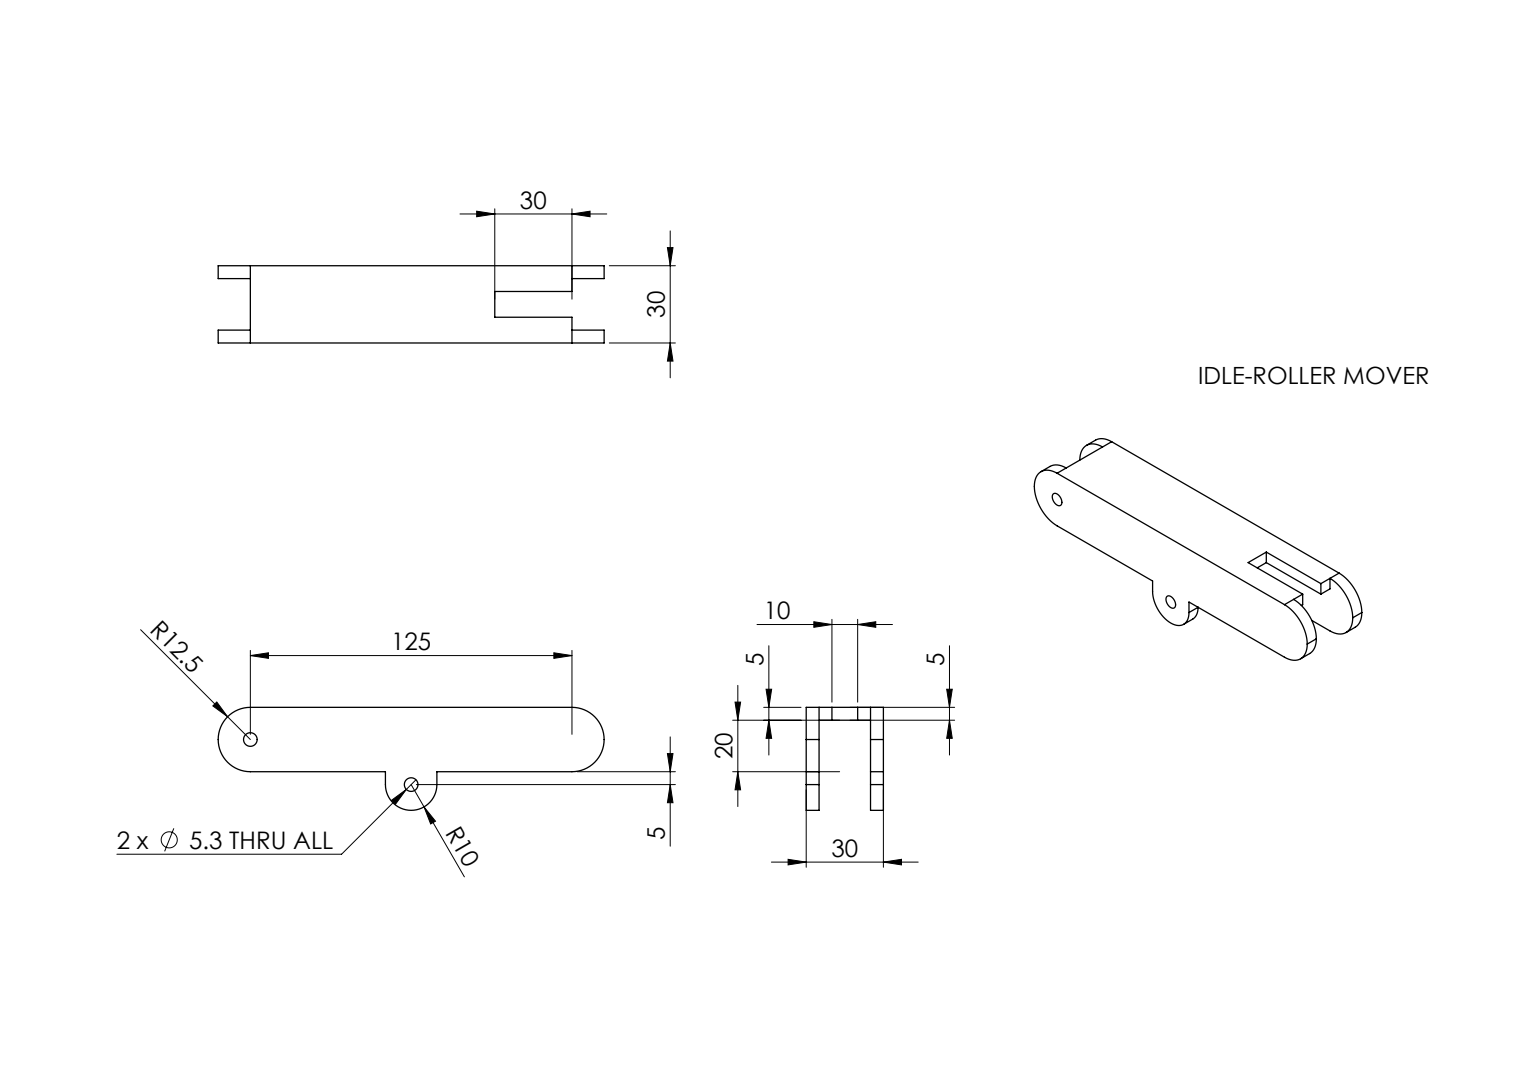
ISO-10303-21;
HEADER;
FILE_DESCRIPTION (('STEP AP214'),
    '1' );
FILE_NAME ('idle-roller mover.step',
    '2026-10-25T07:12:54',
    ( '' ),
    ( '' ),
    'SwSTEP 2.0',
    'SolidWorks 2026',
    '' );
FILE_SCHEMA (( 'AUTOMOTIVE_DESIGN' ));
ENDSEC;

DATA;
#13=CARTESIAN_POINT ( 'NONE',  ( 62.49999999999998579, 40.00000000000001421, 0.000000000000000000 ) ) ;
#53=PLANE ( 'NONE',  #5492 ) ;
#59=AXIS2_PLACEMENT_3D ( 'NONE', #3052, #893, #11418 ) ;
#61=DIRECTION ( 'NONE',  ( -1.000000000000000000, 0.000000000000000000, 0.000000000000000000 ) ) ;
#77=ORIENTED_EDGE ( 'NONE', *, *, #7381, .F. ) ;
#79=ORIENTED_EDGE ( 'NONE', *, *, #8111, .F. ) ;
#81=EDGE_CURVE ( 'NONE', #6144, #12887, #9290, .T. ) ;
#85=DIRECTION ( 'NONE',  ( 1.000000000000000000, -0.000000000000000000, 0.000000000000000000 ) ) ;
#94=ADVANCED_FACE ( 'NONE', ( #8455 ), #6331, .F. ) ;
#97=ADVANCED_FACE ( 'NONE', ( #1883, #8329, #2085 ), #7362, .T. ) ;
#98=DIRECTION ( 'NONE',  ( 0.000000000000000000, -1.000000000000000000, 0.000000000000000000 ) ) ;
#115=ORIENTED_EDGE ( 'NONE', *, *, #9892, .T. ) ;
#157=ADVANCED_FACE ( 'NONE', ( #8524 ), #11972, .T. ) ;
#164=ORIENTED_EDGE ( 'NONE', *, *, #12600, .T. ) ;
#165=CARTESIAN_POINT ( 'NONE',  ( -9.999999999999996447, 0.000000000000000000, 9.999999999999998224 ) ) ;
#166=ORIENTED_EDGE ( 'NONE', *, *, #5950, .F. ) ;
#173=DIRECTION ( 'NONE',  ( 1.000000000000000000, 0.000000000000000000, 0.000000000000000000 ) ) ;
#177=FACE_OUTER_BOUND ( 'NONE', #6171, .T. ) ;
#178=VERTEX_POINT ( 'NONE', #7689 ) ;
#182=FACE_OUTER_BOUND ( 'NONE', #2923, .T. ) ;
#199=ORIENTED_EDGE ( 'NONE', *, *, #13522, .F. ) ;
#200=CARTESIAN_POINT ( 'NONE',  ( 32.49999999999998579, 40.00000000000001421, -4.999999999999996447 ) ) ;
#212=ORIENTED_EDGE ( 'NONE', *, *, #12682, .T. ) ;
#219=FACE_BOUND ( 'NONE', #1402, .T. ) ;
#220=CARTESIAN_POINT ( 'NONE',  ( -74.99999999999997158, 20.00000000000001421, 15.00000000000000000 ) ) ;
#234=ORIENTED_EDGE ( 'NONE', *, *, #2081, .F. ) ;
#244=DIRECTION ( 'NONE',  ( 0.000000000000000000, -0.000000000000000000, 1.000000000000000000 ) ) ;
#245=VERTEX_POINT ( 'NONE', #4504 ) ;
#247=ORIENTED_EDGE ( 'NONE', *, *, #4058, .T. ) ;
#256=AXIS2_PLACEMENT_3D ( 'NONE', #2457, #12077, #2596 ) ;
#262=AXIS2_PLACEMENT_3D ( 'NONE', #4018, #5829, #10026 ) ;
#266=ADVANCED_FACE ( 'NONE', ( #8732 ), #10661, .F. ) ;
#267=EDGE_CURVE ( 'NONE', #10003, #9221, #8792, .T. ) ;
#304=CARTESIAN_POINT ( 'NONE',  ( 9.999999999999994671, 20.00000000000001421, 15.00000000000000000 ) ) ;
#311=ORIENTED_EDGE ( 'NONE', *, *, #8812, .T. ) ;
#313=ORIENTED_EDGE ( 'NONE', *, *, #6610, .T. ) ;
#319=CARTESIAN_POINT ( 'NONE',  ( -9.999999999999994671, 20.00000000000001421, -9.999999999999998224 ) ) ;
#343=EDGE_CURVE ( 'NONE', #10107, #1320, #11620, .T. ) ;
#345=VERTEX_POINT ( 'NONE', #12614 ) ;
#351=CARTESIAN_POINT ( 'NONE',  ( -74.99999999999997158, 45.00000000000001421, 15.00000000000000000 ) ) ;
#358=CIRCLE ( 'NONE', #5021, 12.49999999999999645 ) ;
#380=CARTESIAN_POINT ( 'NONE',  ( -9.999999999999994671, 20.00000000000001421, -15.00000000000000000 ) ) ;
#389=ORIENTED_EDGE ( 'NONE', *, *, #8812, .F. ) ;
#390=ORIENTED_EDGE ( 'NONE', *, *, #9083, .T. ) ;
#408=VERTEX_POINT ( 'NONE', #12548 ) ;
#409=DIRECTION ( 'NONE',  ( -0.000000000000000000, -0.000000000000000000, 1.000000000000000000 ) ) ;
#430=AXIS2_PLACEMENT_3D ( 'NONE', #5828, #10990, #3471 ) ;
#441=ORIENTED_EDGE ( 'NONE', *, *, #10942, .F. ) ;
#463=DIRECTION ( 'NONE',  ( -0.000000000000000000, -0.000000000000000000, 1.000000000000000000 ) ) ;
#468=DIRECTION ( 'NONE',  ( 0.000000000000000000, 1.000000000000000000, 0.000000000000000000 ) ) ;
#474=ORIENTED_EDGE ( 'NONE', *, *, #8307, .F. ) ;
#489=ORIENTED_EDGE ( 'NONE', *, *, #12347, .F. ) ;
#490=VECTOR ( 'NONE', #3038, 1000.000000000000000 ) ;
#499=DIRECTION ( 'NONE',  ( -0.000000000000000000, 0.000000000000000000, -1.000000000000000000 ) ) ;
#502=DIRECTION ( 'NONE',  ( -0.000000000000000000, -0.000000000000000000, 1.000000000000000000 ) ) ;
#516=CARTESIAN_POINT ( 'NONE',  ( 62.49999999999998579, 32.50000000000001421, 9.999999999999998224 ) ) ;
#525=CIRCLE ( 'NONE', #9155, 2.649999999999985700 ) ;
#529=CIRCLE ( 'NONE', #3856, 2.649999999999988809 ) ;
#533=EDGE_CURVE ( 'NONE', #8787, #7994, #6142, .T. ) ;
#548=CARTESIAN_POINT ( 'NONE',  ( 75.00000000000000000, 32.50000000000001421, 15.00000000000000000 ) ) ;
#559=DIRECTION ( 'NONE',  ( -0.000000000000000000, -0.000000000000000000, 1.000000000000000000 ) ) ;
#570=DIRECTION ( 'NONE',  ( -1.000000000000000000, 0.000000000000000000, 0.000000000000000000 ) ) ;
#587=EDGE_CURVE ( 'NONE', #10229, #12054, #9700, .T. ) ;
#590=EDGE_CURVE ( 'NONE', #178, #4538, #10739, .T. ) ;
#603=CARTESIAN_POINT ( 'NONE',  ( 1.925929944387235853E-31, 15.00000000000001599, 15.00000000000000178 ) ) ;
#604=DIRECTION ( 'NONE',  ( 0.000000000000000000, -0.000000000000000000, 1.000000000000000000 ) ) ;
#614=VERTEX_POINT ( 'NONE', #11711 ) ;
#624=CARTESIAN_POINT ( 'NONE',  ( -62.49999999999997158, 20.00000000000001421, -15.00000000000000000 ) ) ;
#632=ORIENTED_EDGE ( 'NONE', *, *, #4500, .T. ) ;
#633=ORIENTED_EDGE ( 'NONE', *, *, #6574, .T. ) ;
#648=STYLED_ITEM ( 'NONE', ( #11200 ), #1529 ) ;
#650=ORIENTED_EDGE ( 'NONE', *, *, #12597, .T. ) ;
#665=ORIENTED_EDGE ( 'NONE', *, *, #7392, .F. ) ;
#673=LINE ( 'NONE', #12175, #10645 ) ;
#675=DIRECTION ( 'NONE',  ( -1.000000000000000000, 0.000000000000000000, 1.224646799147353207E-16 ) ) ;
#681=AXIS2_PLACEMENT_3D ( 'NONE', #3109, #7339, #6931 ) ;
#685=ORIENTED_EDGE ( 'NONE', *, *, #5886, .F. ) ;
#727=CARTESIAN_POINT ( 'NONE',  ( -9.999999999999996447, 0.000000000000000000, -9.999999999999998224 ) ) ;
#740=EDGE_LOOP ( 'NONE', ( #13174, #5500 ) ) ;
#749=DIRECTION ( 'NONE',  ( 1.000000000000000000, 0.000000000000000000, 0.000000000000000000 ) ) ;
#776=DIRECTION ( 'NONE',  ( -0.000000000000000000, -0.000000000000000000, 1.000000000000000000 ) ) ;
#782=VECTOR ( 'NONE', #5023, 1000.000000000000000 ) ;
#787=DIRECTION ( 'NONE',  ( 0.000000000000000000, 0.000000000000000000, -1.000000000000000000 ) ) ;
#827=CYLINDRICAL_SURFACE ( 'NONE', #9755, 12.49999999999999645 ) ;
#833=VECTOR ( 'NONE', #4057, 1000.000000000000000 ) ;
#834=LINE ( 'NONE', #8057, #1573 ) ;
#856=AXIS2_PLACEMENT_3D ( 'NONE', #8158, #2895, #7122 ) ;
#865=CARTESIAN_POINT ( 'NONE',  ( -74.99999999999997158, 45.00000000000001421, -15.00000000000000000 ) ) ;
#867=AXIS2_PLACEMENT_3D ( 'NONE', #12641, #5263, #61 ) ;
#886=( LENGTH_UNIT ( ) NAMED_UNIT ( * ) SI_UNIT ( .MILLI., .METRE. ) );
#888=DIRECTION ( 'NONE',  ( 0.000000000000000000, -0.000000000000000000, 1.000000000000000000 ) ) ;
#893=DIRECTION ( 'NONE',  ( -0.000000000000000000, -0.000000000000000000, 1.000000000000000000 ) ) ;
#899=EDGE_LOOP ( 'NONE', ( #12321, #1610, #650, #2100, #2554, #2982, #11409, #10105, #9169, #11499, #11268, #10678 ) ) ;
#919=VERTEX_POINT ( 'NONE', #5981 ) ;
#932=DIRECTION ( 'NONE',  ( -1.000000000000000000, 0.000000000000000000, 0.000000000000000000 ) ) ;
#945=LINE ( 'NONE', #10290, #2409 ) ;
#960=ADVANCED_FACE ( 'NONE', ( #13302 ), #10599, .F. ) ;
#967=VERTEX_POINT ( 'NONE', #1762 ) ;
#974=AXIS2_PLACEMENT_3D ( 'NONE', #13105, #9180, #2883 ) ;
#975=DIRECTION ( 'NONE',  ( -1.000000000000000000, 0.000000000000000000, 0.000000000000000000 ) ) ;
#994=DIRECTION ( 'NONE',  ( -0.000000000000000000, 1.000000000000000000, -0.000000000000000000 ) ) ;
#1018=ORIENTED_EDGE ( 'NONE', *, *, #3599, .T. ) ;
#1019=VERTEX_POINT ( 'NONE', #5356 ) ;
#1022=ADVANCED_FACE ( 'NONE', ( #3205 ), #12346, .F. ) ;
#1024=LINE ( 'NONE', #865, #1101 ) ;
#1025=CARTESIAN_POINT ( 'NONE',  ( -74.99999999999997158, 32.50000000000001421, 15.00000000000000000 ) ) ;
#1036=EDGE_CURVE ( 'NONE', #7994, #9043, #4309, .T. ) ;
#1040=DIRECTION ( 'NONE',  ( -1.000000000000000000, 0.000000000000000000, 0.000000000000000000 ) ) ;
#1043=DIRECTION ( 'NONE',  ( -0.000000000000000000, -0.000000000000000000, 1.000000000000000000 ) ) ;
#1052=VECTOR ( 'NONE', #6708, 1000.000000000000000 ) ;
#1080=ADVANCED_FACE ( 'NONE', ( #1308 ), #13067, .F. ) ;
#1101=VECTOR ( 'NONE', #4222, 1000.000000000000000 ) ;
#1127=CARTESIAN_POINT ( 'NONE',  ( -65.14999999999996305, 32.50000000000001421, -15.00000000000000000 ) ) ;
#1136=VECTOR ( 'NONE', #2029, 1000.000000000000000 ) ;
#1155=ORIENTED_EDGE ( 'NONE', *, *, #6325, .F. ) ;
#1159=LINE ( 'NONE', #4355, #7189 ) ;
#1172=DIRECTION ( 'NONE',  ( 0.000000000000000000, 1.000000000000000000, 0.000000000000000000 ) ) ;
#1195=ADVANCED_FACE ( 'NONE', ( #2914 ), #12926, .T. ) ;
#1200=EDGE_CURVE ( 'NONE', #13024, #10854, #10028, .T. ) ;
#1208=ORIENTED_EDGE ( 'NONE', *, *, #8540, .F. ) ;
#1210=CIRCLE ( 'NONE', #4730, 12.49999999999999645 ) ;
#1238=CARTESIAN_POINT ( 'NONE',  ( -9.999999999999994671, 20.00000000000001421, 15.00000000000000000 ) ) ;
#1272=EDGE_CURVE ( 'NONE', #4573, #7186, #10236, .T. ) ;
#1279=CARTESIAN_POINT ( 'NONE',  ( 10.00000000000000000, 25.00000000000001776, 15.00000000000000000 ) ) ;
#1289=DIRECTION ( 'NONE',  ( -1.000000000000000000, 1.110223024625156935E-15, 0.000000000000000000 ) ) ;
#1303=ORIENTED_EDGE ( 'NONE', *, *, #5017, .T. ) ;
#1308=FACE_OUTER_BOUND ( 'NONE', #9255, .T. ) ;
#1320=VERTEX_POINT ( 'NONE', #9211 ) ;
#1323=EDGE_CURVE ( 'NONE', #11747, #7759, #358, .T. ) ;
#1335=VECTOR ( 'NONE', #1410, 1000.000000000000000 ) ;
#1337=DIRECTION ( 'NONE',  ( -1.000000000000000000, 0.000000000000000000, 0.000000000000000000 ) ) ;
#1342=DIRECTION ( 'NONE',  ( -1.000000000000000000, 0.000000000000000000, 0.000000000000000000 ) ) ;
#1356=ORIENTED_EDGE ( 'NONE', *, *, #8047, .T. ) ;
#1363=CARTESIAN_POINT ( 'NONE',  ( -65.14999999999996305, 32.50000000000001421, 15.00000000000000178 ) ) ;
#1376=LINE ( 'NONE', #1238, #2906 ) ;
#1386=VERTEX_POINT ( 'NONE', #1025 ) ;
#1402=EDGE_LOOP ( 'NONE', ( #7892, #3977 ) ) ;
#1410=DIRECTION ( 'NONE',  ( -0.000000000000000000, -0.000000000000000000, -1.000000000000000000 ) ) ;
#1432=FACE_OUTER_BOUND ( 'NONE', #10283, .T. ) ;
#1440=ORIENTED_EDGE ( 'NONE', *, *, #7392, .T. ) ;
#1443=CYLINDRICAL_SURFACE ( 'NONE', #12538, 12.49999999999999645 ) ;
#1471=ORIENTED_EDGE ( 'NONE', *, *, #7707, .F. ) ;
#1475=CARTESIAN_POINT ( 'NONE',  ( 62.49999999999998579, 45.00000000000001421, 15.00000000000000000 ) ) ;
#1491=AXIS2_PLACEMENT_3D ( 'NONE', #7044, #8152, #5045 ) ;
#1516=AXIS2_PLACEMENT_3D ( 'NONE', #9631, #7302, #11509 ) ;
#1529=ADVANCED_BREP_SHAPE_REPRESENTATION ( '', ( #10251, #430 ), #10167 ) ;
#1545=CARTESIAN_POINT ( 'NONE',  ( 62.50000000000000000, 32.50000000000001421, -15.00000000000000000 ) ) ;
#1552=CARTESIAN_POINT ( 'NONE',  ( 62.50000000000000000, 20.00000000000001421, 15.00000000000000000 ) ) ;
#1561=LINE ( 'NONE', #6772, #1866 ) ;
#1562=VECTOR ( 'NONE', #12045, 1000.000000000000000 ) ;
#1564=VECTOR ( 'NONE', #4461, 1000.000000000000000 ) ;
#1573=VECTOR ( 'NONE', #6134, 1000.000000000000000 ) ;
#1579=CARTESIAN_POINT ( 'NONE',  ( 32.49999999999998579, 45.00000000000001421, -4.999999999999996447 ) ) ;
#1583=CARTESIAN_POINT ( 'NONE',  ( -74.99999999999997158, 20.00000000000001421, -15.00000000000000000 ) ) ;
#1602=LINE ( 'NONE', #12470, #5242 ) ;
#1610=ORIENTED_EDGE ( 'NONE', *, *, #10696, .T. ) ;
#1614=DIRECTION ( 'NONE',  ( -0.000000000000000000, -0.000000000000000000, 1.000000000000000000 ) ) ;
#1618=ADVANCED_FACE ( 'NONE', ( #3928 ), #9260, .F. ) ;
#1632=ORIENTED_EDGE ( 'NONE', *, *, #12015, .T. ) ;
#1642=FACE_BOUND ( 'NONE', #9538, .T. ) ;
#1651=CARTESIAN_POINT ( 'NONE',  ( -59.84999999999998721, 32.50000000000001421, -9.999999999999998224 ) ) ;
#1654=CARTESIAN_POINT ( 'NONE',  ( 62.50000000000000000, 32.50000000000001421, 9.999999999999998224 ) ) ;
#1659=DIRECTION ( 'NONE',  ( 0.000000000000000000, 0.000000000000000000, -1.000000000000000000 ) ) ;
#1668=CARTESIAN_POINT ( 'NONE',  ( -9.999999999999994671, 20.00000000000001421, 15.00000000000000000 ) ) ;
#1673=FACE_OUTER_BOUND ( 'NONE', #12257, .T. ) ;
#1684=DIRECTION ( 'NONE',  ( 0.000000000000000000, 0.000000000000000000, 1.000000000000000000 ) ) ;
#1721=SURFACE_STYLE_USAGE ( .BOTH. , #9137 ) ;
#1734=ORIENTED_EDGE ( 'NONE', *, *, #5860, .F. ) ;
#1737=ORIENTED_EDGE ( 'NONE', *, *, #5970, .T. ) ;
#1762=CARTESIAN_POINT ( 'NONE',  ( 62.49999999999998579, 45.00000000000001421, -5.000000000000000000 ) ) ;
#1775=EDGE_CURVE ( 'NONE', #11894, #614, #6502, .T. ) ;
#1794=LINE ( 'NONE', #2985, #6464 ) ;
#1803=DIRECTION ( 'NONE',  ( -1.000000000000000000, 0.000000000000000000, 0.000000000000000000 ) ) ;
#1830=CARTESIAN_POINT ( 'NONE',  ( -74.99999999999997158, 32.50000000000001421, 15.00000000000000000 ) ) ;
#1854=LINE ( 'NONE', #6168, #3384 ) ;
#1866=VECTOR ( 'NONE', #4768, 1000.000000000000000 ) ;
#1883=FACE_BOUND ( 'NONE', #13295, .T. ) ;
#1905=CARTESIAN_POINT ( 'NONE',  ( 62.49999999999998579, 5.000000000000018652, -5.000000000000000000 ) ) ;
#1932=CARTESIAN_POINT ( 'NONE',  ( 1.925929944387235853E-31, 15.00000000000001599, 15.00000000000000000 ) ) ;
#1939=CARTESIAN_POINT ( 'NONE',  ( 1.925929944387235853E-31, 15.00000000000001599, 9.999999999999998224 ) ) ;
#1959=DIRECTION ( 'NONE',  ( 0.000000000000000000, 0.000000000000000000, -1.000000000000000000 ) ) ;
#1974=LINE ( 'NONE', #1830, #6444 ) ;
#1976=CIRCLE ( 'NONE', #1516, 12.49999999999999645 ) ;
#1983=EDGE_LOOP ( 'NONE', ( #2851, #3400, #11674, #11892 ) ) ;
#2005=CIRCLE ( 'NONE', #867, 12.49999999999999645 ) ;
#2029=DIRECTION ( 'NONE',  ( 0.000000000000000000, 0.000000000000000000, -1.000000000000000000 ) ) ;
#2030=DIRECTION ( 'NONE',  ( -1.000000000000000000, 0.000000000000000000, 0.000000000000000000 ) ) ;
#2052=ADVANCED_FACE ( 'NONE', ( #9106 ), #3508, .T. ) ;
#2053=AXIS2_PLACEMENT_3D ( 'NONE', #7555, #1172, #5423 ) ;
#2057=CARTESIAN_POINT ( 'NONE',  ( -74.99999999999997158, 40.00000000000001421, 5.000000000000018652 ) ) ;
#2069=CARTESIAN_POINT ( 'NONE',  ( -2.649999999999988365, 15.00000000000001599, 9.999999999999998224 ) ) ;
#2081=EDGE_CURVE ( 'NONE', #10697, #3166, #4244, .T. ) ;
#2085=FACE_OUTER_BOUND ( 'NONE', #6497, .T. ) ;
#2100=ORIENTED_EDGE ( 'NONE', *, *, #8511, .F. ) ;
#2111=CARTESIAN_POINT ( 'NONE',  ( 0.000000000000000000, 40.00000000000001421, -9.999999999999998224 ) ) ;
#2135=CYLINDRICAL_SURFACE ( 'NONE', #3362, 2.649999999999985700 ) ;
#2197=AXIS2_PLACEMENT_3D ( 'NONE', #5465, #11941, #6634 ) ;
#2212=EDGE_CURVE ( 'NONE', #6833, #12476, #6611, .T. ) ;
#2217=ADVANCED_FACE ( 'NONE', ( #10689 ), #8818, .F. ) ;
#2218=LINE ( 'NONE', #3202, #2513 ) ;
#2219=CARTESIAN_POINT ( 'NONE',  ( 62.49999999999998579, 45.00000000000001421, -9.999999999999998224 ) ) ;
#2222=CARTESIAN_POINT ( 'NONE',  ( -74.99999999999997158, 32.50000000000001421, -15.00000000000000000 ) ) ;
#2229=LINE ( 'NONE', #6473, #11363 ) ;
#2231=DIRECTION ( 'NONE',  ( 0.000000000000000000, 0.000000000000000000, -1.000000000000000000 ) ) ;
#2235=PRODUCT ( 'idle-roller mover', 'idle-roller mover', '', ( #2933 ) ) ;
#2255=AXIS2_PLACEMENT_3D ( 'NONE', #1939, #13474, #1803 ) ;
#2257=EDGE_CURVE ( 'NONE', #1320, #10476, #11856, .T. ) ;
#2279=ORIENTED_EDGE ( 'NONE', *, *, #2720, .T. ) ;
#2302=VECTOR ( 'NONE', #6827, 1000.000000000000000 ) ;
#2334=CARTESIAN_POINT ( 'NONE',  ( 62.50000000000000000, 32.50000000000001421, 15.00000000000000000 ) ) ;
#2373=( GEOMETRIC_REPRESENTATION_CONTEXT ( 3 ) GLOBAL_UNCERTAINTY_ASSIGNED_CONTEXT ( ( #8960 ) ) GLOBAL_UNIT_ASSIGNED_CONTEXT ( ( #2560, #9691, #5550 ) ) REPRESENTATION_CONTEXT ( 'NONE', 'WORKASPACE' ) );
#2388=CARTESIAN_POINT ( 'NONE',  ( -62.49999999999997158, 32.50000000000001421, 15.00000000000000000 ) ) ;
#2399=ORIENTED_EDGE ( 'NONE', *, *, #9923, .F. ) ;
#2402=ORIENTED_EDGE ( 'NONE', *, *, #8307, .T. ) ;
#2409=VECTOR ( 'NONE', #4142, 1000.000000000000000 ) ;
#2413=AXIS2_PLACEMENT_3D ( 'NONE', #13508, #7430, #10344 ) ;
#2447=CYLINDRICAL_SURFACE ( 'NONE', #13079, 12.49999999999999645 ) ;
#2450=AXIS2_PLACEMENT_3D ( 'NONE', #4261, #6543, #11529 ) ;
#2457=CARTESIAN_POINT ( 'NONE',  ( -62.49999999999997158, 32.50000000000001421, 15.00000000000000000 ) ) ;
#2459=CIRCLE ( 'NONE', #11291, 2.649999999999985700 ) ;
#2475=VECTOR ( 'NONE', #468, 1000.000000000000000 ) ;
#2493=FACE_OUTER_BOUND ( 'NONE', #8185, .T. ) ;
#2501=CARTESIAN_POINT ( 'NONE',  ( 32.49999999999998579, 5.000000000000018652, 5.000000000000003553 ) ) ;
#2513=VECTOR ( 'NONE', #8590, 1000.000000000000000 ) ;
#2520=VECTOR ( 'NONE', #502, 1000.000000000000000 ) ;
#2523=PLANE ( 'NONE',  #2611 ) ;
#2524=CIRCLE ( 'NONE', #6949, 12.49999999999999645 ) ;
#2528=DIRECTION ( 'NONE',  ( -1.000000000000000000, 0.000000000000000000, 0.000000000000000000 ) ) ;
#2538=EDGE_LOOP ( 'NONE', ( #4728, #1208, #10269, #10720 ) ) ;
#2544=EDGE_CURVE ( 'NONE', #614, #408, #1602, .T. ) ;
#2551=CARTESIAN_POINT ( 'NONE',  ( 1.925929944387235853E-31, 15.00000000000001599, 15.00000000000000000 ) ) ;
#2554=ORIENTED_EDGE ( 'NONE', *, *, #3984, .T. ) ;
#2560=( LENGTH_UNIT ( ) NAMED_UNIT ( * ) SI_UNIT ( .MILLI., .METRE. ) );
#2564=DIRECTION ( 'NONE',  ( -0.000000000000000000, -0.000000000000000000, 1.000000000000000000 ) ) ;
#2592=DIRECTION ( 'NONE',  ( -1.000000000000000000, 0.000000000000000000, 0.000000000000000000 ) ) ;
#2596=DIRECTION ( 'NONE',  ( -1.000000000000000000, 0.000000000000000000, 0.000000000000000000 ) ) ;
#2599=LINE ( 'NONE', #1552, #2302 ) ;
#2611=AXIS2_PLACEMENT_3D ( 'NONE', #4678, #13160, #9921 ) ;
#2617=CARTESIAN_POINT ( 'NONE',  ( -62.49999999999997158, 45.00000000000001421, 9.999999999999998224 ) ) ;
#2625=ORIENTED_EDGE ( 'NONE', *, *, #9989, .F. ) ;
#2626=VECTOR ( 'NONE', #10473, 1000.000000000000000 ) ;
#2628=FACE_OUTER_BOUND ( 'NONE', #13159, .T. ) ;
#2636=CARTESIAN_POINT ( 'NONE',  ( -62.49999999999997158, 32.50000000000001421, -9.999999999999998224 ) ) ;
#2638=EDGE_CURVE ( 'NONE', #1386, #9920, #9498, .T. ) ;
#2641=EDGE_CURVE ( 'NONE', #10476, #6120, #3235, .T. ) ;
#2642=ORIENTED_EDGE ( 'NONE', *, *, #2257, .F. ) ;
#2657=CYLINDRICAL_SURFACE ( 'NONE', #12026, 12.49999999999999645 ) ;
#2668=DIRECTION ( 'NONE',  ( -0.000000000000000000, -0.000000000000000000, 1.000000000000000000 ) ) ;
#2671=LINE ( 'NONE', #13374, #13561 ) ;
#2675=ADVANCED_FACE ( 'NONE', ( #9369 ), #7371, .F. ) ;
#2678=EDGE_LOOP ( 'NONE', ( #12084, #5636, #1440, #4102 ) ) ;
#2682=AXIS2_PLACEMENT_3D ( 'NONE', #10460, #10393, #4172 ) ;
#2690=LINE ( 'NONE', #2617, #2475 ) ;
#2693=AXIS2_PLACEMENT_3D ( 'NONE', #13356, #10259, #12398 ) ;
#2699=FILL_AREA_STYLE ('',( #9275 ) ) ;
#2701=CYLINDRICAL_SURFACE ( 'NONE', #12377, 12.49999999999999645 ) ;
#2706=VECTOR ( 'NONE', #6733, 1000.000000000000000 ) ;
#2707=PLANE ( 'NONE',  #681 ) ;
#2710=AXIS2_PLACEMENT_3D ( 'NONE', #13622, #8391, #3128 ) ;
#2718=CARTESIAN_POINT ( 'NONE',  ( -62.49999999999997158, 32.50000000000001421, 15.00000000000000000 ) ) ;
#2720=EDGE_CURVE ( 'NONE', #4781, #9621, #4114, .T. ) ;
#2731=ORIENTED_EDGE ( 'NONE', *, *, #4598, .F. ) ;
#2735=CARTESIAN_POINT ( 'NONE',  ( 1.925929944387235853E-31, 15.00000000000001599, 15.00000000000000000 ) ) ;
#2737=DIRECTION ( 'NONE',  ( 0.000000000000000000, 0.000000000000000000, -1.000000000000000000 ) ) ;
#2745=CARTESIAN_POINT ( 'NONE',  ( -9.999999999999998224, 15.00000000000001776, 15.00000000000000000 ) ) ;
#2751=VECTOR ( 'NONE', #9258, 1000.000000000000000 ) ;
#2756=DIRECTION ( 'NONE',  ( 1.000000000000000000, 0.000000000000000000, 0.000000000000000000 ) ) ;
#2757=AXIS2_PLACEMENT_3D ( 'NONE', #12688, #13511, #3023 ) ;
#2764=DIRECTION ( 'NONE',  ( 0.000000000000000000, 0.000000000000000000, -1.000000000000000000 ) ) ;
#2774=( NAMED_UNIT ( * ) SI_UNIT ( $, .STERADIAN. ) SOLID_ANGLE_UNIT ( ) );
#2802=DIRECTION ( 'NONE',  ( 0.000000000000000000, -0.000000000000000000, 1.000000000000000000 ) ) ;
#2815=CYLINDRICAL_SURFACE ( 'NONE', #4981, 2.649999999999988365 ) ;
#2818=EDGE_LOOP ( 'NONE', ( #8993, #7956, #9062, #9327 ) ) ;
#2823=PLANE ( 'NONE',  #1491 ) ;
#2828=STYLED_ITEM('',(#13698),#10251);
#2832=DIRECTION ( 'NONE',  ( 1.000000000000000000, 0.000000000000000000, 0.000000000000000000 ) ) ;
#2835=ORIENTED_EDGE ( 'NONE', *, *, #9989, .T. ) ;
#2836=APPLICATION_CONTEXT ( 'automotive_design' ) ;
#2841=( NAMED_UNIT ( * ) PLANE_ANGLE_UNIT ( ) SI_UNIT ( $, .RADIAN. ) );
#2851=ORIENTED_EDGE ( 'NONE', *, *, #267, .F. ) ;
#2863=LINE ( 'NONE', #9298, #13057 ) ;
#2866=LINE ( 'NONE', #10263, #12636 ) ;
#2871=ORIENTED_EDGE ( 'NONE', *, *, #6489, .F. ) ;
#2873=ORIENTED_EDGE ( 'NONE', *, *, #4058, .F. ) ;
#2883=DIRECTION ( 'NONE',  ( -1.000000000000000000, 0.000000000000000000, 1.224646799147353207E-16 ) ) ;
#2895=DIRECTION ( 'NONE',  ( 1.000000000000000000, 0.000000000000000000, -0.000000000000000000 ) ) ;
#2906=VECTOR ( 'NONE', #9763, 1000.000000000000000 ) ;
#2907=VERTEX_POINT ( 'NONE', #11906 ) ;
#2910=( NAMED_UNIT ( * ) PLANE_ANGLE_UNIT ( ) SI_UNIT ( $, .RADIAN. ) );
#2914=FACE_OUTER_BOUND ( 'NONE', #899, .T. ) ;
#2923=EDGE_LOOP ( 'NONE', ( #166, #1303, #5281, #9689 ) ) ;
#2931=DIRECTION ( 'NONE',  ( 1.000000000000000000, 0.000000000000000000, 0.000000000000000000 ) ) ;
#2933=PRODUCT_CONTEXT ( 'NONE', #2836, 'mechanical' ) ;
#2963=ORIENTED_EDGE ( 'NONE', *, *, #2212, .F. ) ;
#2967=DIRECTION ( 'NONE',  ( -1.224646799147353207E-16, 0.000000000000000000, -1.000000000000000000 ) ) ;
#2973=EDGE_CURVE ( 'NONE', #12054, #614, #3164, .T. ) ;
#2975=EDGE_CURVE ( 'NONE', #7759, #10697, #5977, .T. ) ;
#2982=ORIENTED_EDGE ( 'NONE', *, *, #2544, .T. ) ;
#2984=VECTOR ( 'NONE', #5047, 1000.000000000000000 ) ;
#2985=CARTESIAN_POINT ( 'NONE',  ( 2.649999999999988365, 15.00000000000001599, 15.00000000000000000 ) ) ;
#2999=DIRECTION ( 'NONE',  ( -0.000000000000000000, -0.000000000000000000, 1.000000000000000000 ) ) ;
#3014=ORIENTED_EDGE ( 'NONE', *, *, #7162, .F. ) ;
#3023=DIRECTION ( 'NONE',  ( -1.000000000000000000, 0.000000000000000000, 0.000000000000000000 ) ) ;
#3038=DIRECTION ( 'NONE',  ( -0.000000000000000000, 0.000000000000000000, 1.000000000000000000 ) ) ;
#3042=ORIENTED_EDGE ( 'NONE', *, *, #3183, .F. ) ;
#3046=DIRECTION ( 'NONE',  ( 1.000000000000000000, 0.000000000000000000, 0.000000000000000000 ) ) ;
#3047=CARTESIAN_POINT ( 'NONE',  ( -62.49999999999997158, 32.50000000000001421, -15.00000000000000000 ) ) ;
#3052=CARTESIAN_POINT ( 'NONE',  ( -62.49999999999997158, 32.50000000000001421, 15.00000000000000178 ) ) ;
#3055=ORIENTED_EDGE ( 'NONE', *, *, #3685, .T. ) ;
#3059=ORIENTED_EDGE ( 'NONE', *, *, #5886, .T. ) ;
#3080=CIRCLE ( 'NONE', #10790, 12.49999999999999645 ) ;
#3084=VECTOR ( 'NONE', #98, 1000.000000000000000 ) ;
#3089=CARTESIAN_POINT ( 'NONE',  ( -74.99999999999997158, 32.50000000000001421, 9.999999999999998224 ) ) ;
#3099=LINE ( 'NONE', #2057, #2751 ) ;
#3109=CARTESIAN_POINT ( 'NONE',  ( 32.49999999999998579, 5.000000000000018652, 5.000000000000003553 ) ) ;
#3114=DIRECTION ( 'NONE',  ( -1.000000000000000000, 0.000000000000000000, 0.000000000000000000 ) ) ;
#3128=DIRECTION ( 'NONE',  ( 0.000000000000000000, 0.000000000000000000, 1.000000000000000000 ) ) ;
#3153=EDGE_CURVE ( 'NONE', #919, #10854, #8801, .T. ) ;
#3164=CIRCLE ( 'NONE', #10873, 12.49999999999999645 ) ;
#3166=VERTEX_POINT ( 'NONE', #6186 ) ;
#3183=EDGE_CURVE ( 'NONE', #10299, #9221, #11093, .T. ) ;
#3197=EDGE_LOOP ( 'NONE', ( #5861, #685, #4051, #1018 ) ) ;
#3202=CARTESIAN_POINT ( 'NONE',  ( 32.49999999999998579, 45.00000000000001421, 5.000000000000003553 ) ) ;
#3205=FACE_OUTER_BOUND ( 'NONE', #10609, .T. ) ;
#3217=EDGE_CURVE ( 'NONE', #9824, #11777, #11758, .T. ) ;
#3220=ORIENTED_EDGE ( 'NONE', *, *, #587, .F. ) ;
#3235=CIRCLE ( 'NONE', #3672, 2.649999999999985700 ) ;
#3237=EDGE_LOOP ( 'NONE', ( #3059, #7039, #9360, #8788 ) ) ;
#3252=ORIENTED_EDGE ( 'NONE', *, *, #12347, .T. ) ;
#3253=ORIENTED_EDGE ( 'NONE', *, *, #3692, .T. ) ;
#3272=DIRECTION ( 'NONE',  ( 1.000000000000000000, 0.000000000000000000, 0.000000000000000000 ) ) ;
#3283=VECTOR ( 'NONE', #11253, 1000.000000000000000 ) ;
#3296=VERTEX_POINT ( 'NONE', #8519 ) ;
#3312=PLANE ( 'NONE',  #7041 ) ;
#3336=CARTESIAN_POINT ( 'NONE',  ( 62.49999999999998579, 20.00000000000001421, -15.00000000000000000 ) ) ;
#3362=AXIS2_PLACEMENT_3D ( 'NONE', #2388, #12896, #3046 ) ;
#3384=VECTOR ( 'NONE', #8164, 1000.000000000000000 ) ;
#3398=EDGE_LOOP ( 'NONE', ( #13656, #2279, #115, #3907 ) ) ;
#3400=ORIENTED_EDGE ( 'NONE', *, *, #5195, .T. ) ;
#3418=CIRCLE ( 'NONE', #2757, 2.649999999999988365 ) ;
#3435=UNCERTAINTY_MEASURE_WITH_UNIT (LENGTH_MEASURE( 1.000000000000000082E-05 ), #886, 'distance_accuracy_value', 'NONE');
#3436=ORIENTED_EDGE ( 'NONE', *, *, #10318, .T. ) ;
#3441=FACE_OUTER_BOUND ( 'NONE', #2818, .T. ) ;
#3452=DIRECTION ( 'NONE',  ( -0.000000000000000000, -0.000000000000000000, 1.000000000000000000 ) ) ;
#3453=VECTOR ( 'NONE', #7233, 1000.000000000000000 ) ;
#3454=EDGE_CURVE ( 'NONE', #13259, #408, #2690, .T. ) ;
#3469=CARTESIAN_POINT ( 'NONE',  ( -65.14999999999996305, 32.50000000000001421, 15.00000000000000000 ) ) ;
#3471=DIRECTION ( 'NONE',  ( 1.000000000000000000, 0.000000000000000000, 0.000000000000000000 ) ) ;
#3481=ORIENTED_EDGE ( 'NONE', *, *, #10596, .F. ) ;
#3486=DIRECTION ( 'NONE',  ( 0.000000000000000000, 0.000000000000000000, 1.000000000000000000 ) ) ;
#3488=ADVANCED_FACE ( 'NONE', ( #5819 ), #12036, .F. ) ;
#3497=ORIENTED_EDGE ( 'NONE', *, *, #1323, .T. ) ;
#3501=FACE_BOUND ( 'NONE', #10771, .T. ) ;
#3503=DIRECTION ( 'NONE',  ( -0.000000000000000000, 0.000000000000000000, -1.000000000000000000 ) ) ;
#3508=CYLINDRICAL_SURFACE ( 'NONE', #256, 12.49999999999999645 ) ;
#3518=ORIENTED_EDGE ( 'NONE', *, *, #2975, .T. ) ;
#3533=ORIENTED_EDGE ( 'NONE', *, *, #6620, .F. ) ;
#3536=DIRECTION ( 'NONE',  ( -0.000000000000000000, -0.000000000000000000, -1.000000000000000000 ) ) ;
#3548=CIRCLE ( 'NONE', #3761, 2.649999999999985700 ) ;
#3549=ORIENTED_EDGE ( 'NONE', *, *, #4404, .F. ) ;
#3567=ADVANCED_FACE ( 'NONE', ( #1642, #5885, #1432 ), #10085, .F. ) ;
#3582=VECTOR ( 'NONE', #7232, 1000.000000000000000 ) ;
#3599=EDGE_CURVE ( 'NONE', #12887, #7922, #12984, .T. ) ;
#3604=ORIENTED_EDGE ( 'NONE', *, *, #533, .T. ) ;
#3610=CARTESIAN_POINT ( 'NONE',  ( 62.49999999999998579, 45.00000000000001421, 15.00000000000000000 ) ) ;
#3620=ORIENTED_EDGE ( 'NONE', *, *, #3599, .F. ) ;
#3622=AXIS2_PLACEMENT_3D ( 'NONE', #1545, #5865, #570 ) ;
#3625=EDGE_CURVE ( 'NONE', #7328, #9621, #11769, .T. ) ;
#3657=CARTESIAN_POINT ( 'NONE',  ( 1.925929944387235853E-31, 15.00000000000001599, -15.00000000000000000 ) ) ;
#3672=AXIS2_PLACEMENT_3D ( 'NONE', #5296, #11371, #2030 ) ;
#3685=EDGE_CURVE ( 'NONE', #10142, #12202, #1854, .T. ) ;
#3692=EDGE_CURVE ( 'NONE', #11894, #13259, #13320, .T. ) ;
#3701=VERTEX_POINT ( 'NONE', #6030 ) ;
#3709=LINE ( 'NONE', #7933, #4206 ) ;
#3737=AXIS2_PLACEMENT_3D ( 'NONE', #8542, #2231, #6539 ) ;
#3738=LINE ( 'NONE', #8030, #10767 ) ;
#3740=DIRECTION ( 'NONE',  ( -0.000000000000000000, -0.000000000000000000, 1.000000000000000000 ) ) ;
#3761=AXIS2_PLACEMENT_3D ( 'NONE', #7833, #4577, #7763 ) ;
#3768=ORIENTED_EDGE ( 'NONE', *, *, #12355, .T. ) ;
#3801=ADVANCED_FACE ( 'NONE', ( #177 ), #2447, .T. ) ;
#3803=AXIS2_PLACEMENT_3D ( 'NONE', #1932, #10826, #1342 ) ;
#3808=ORIENTED_EDGE ( 'NONE', *, *, #8511, .T. ) ;
#3842=DIRECTION ( 'NONE',  ( -1.000000000000000000, 0.000000000000000000, 0.000000000000000000 ) ) ;
#3846=AXIS2_PLACEMENT_3D ( 'NONE', #10322, #4871, #3892 ) ;
#3856=AXIS2_PLACEMENT_3D ( 'NONE', #3657, #10077, #2756 ) ;
#3879=CARTESIAN_POINT ( 'NONE',  ( 62.49999999999998579, 32.50000000000001421, 15.00000000000000000 ) ) ;
#3892=DIRECTION ( 'NONE',  ( -1.000000000000000000, 0.000000000000000000, 0.000000000000000000 ) ) ;
#3897=SHAPE_REPRESENTATION ( 'idle-roller mover', ( #430 ), #10167 ) ;
#3907=ORIENTED_EDGE ( 'NONE', *, *, #12945, .T. ) ;
#3917=CARTESIAN_POINT ( 'NONE',  ( -9.999999999999998224, 15.00000000000001776, 9.999999999999998224 ) ) ;
#3923=FACE_OUTER_BOUND ( 'NONE', #6975, .T. ) ;
#3928=FACE_OUTER_BOUND ( 'NONE', #3237, .T. ) ;
#3931=VECTOR ( 'NONE', #4575, 1000.000000000000000 ) ;
#3938=ORIENTED_EDGE ( 'NONE', *, *, #11678, .F. ) ;
#3972=DIRECTION ( 'NONE',  ( 1.000000000000000000, -0.000000000000000000, 0.000000000000000000 ) ) ;
#3977=ORIENTED_EDGE ( 'NONE', *, *, #343, .T. ) ;
#3984=EDGE_CURVE ( 'NONE', #4066, #614, #9982, .T. ) ;
#3986=CARTESIAN_POINT ( 'NONE',  ( -65.14999999999996305, 32.50000000000001421, 9.999999999999998224 ) ) ;
#3997=ORIENTED_EDGE ( 'NONE', *, *, #12109, .T. ) ;
#3998=CARTESIAN_POINT ( 'NONE',  ( 75.00000000000000000, 32.50000000000001421, 15.00000000000000000 ) ) ;
#4018=CARTESIAN_POINT ( 'NONE',  ( 62.50000000000000000, 32.50000000000001421, 15.00000000000000000 ) ) ;
#4042=DIRECTION ( 'NONE',  ( 1.000000000000000000, 0.000000000000000000, 0.000000000000000000 ) ) ;
#4043=CARTESIAN_POINT ( 'NONE',  ( 10.00000000000000000, 15.00000000000001776, 15.00000000000000000 ) ) ;
#4051=ORIENTED_EDGE ( 'NONE', *, *, #81, .T. ) ;
#4057=DIRECTION ( 'NONE',  ( -0.000000000000000000, -0.000000000000000000, 1.000000000000000000 ) ) ;
#4058=EDGE_CURVE ( 'NONE', #9221, #10299, #525, .T. ) ;
#4066=VERTEX_POINT ( 'NONE', #5788 ) ;
#4102=ORIENTED_EDGE ( 'NONE', *, *, #12746, .F. ) ;
#4114=LINE ( 'NONE', #4043, #782 ) ;
#4125=PRODUCT_DEFINITION_SHAPE ( 'NONE', 'NONE',  #10465 ) ;
#4142=DIRECTION ( 'NONE',  ( 0.000000000000000000, 1.000000000000000000, 0.000000000000000000 ) ) ;
#4148=ADVANCED_FACE ( 'NONE', ( #12201 ), #2657, .T. ) ;
#4167=ORIENTED_EDGE ( 'NONE', *, *, #5970, .F. ) ;
#4172=DIRECTION ( 'NONE',  ( -0.000000000000000000, 0.000000000000000000, -1.000000000000000000 ) ) ;
#4178=LINE ( 'NONE', #8402, #9973 ) ;
#4198=CARTESIAN_POINT ( 'NONE',  ( -62.49999999999997158, 32.50000000000001421, 9.999999999999998224 ) ) ;
#4202=EDGE_CURVE ( 'NONE', #6833, #11747, #9373, .T. ) ;
#4206=VECTOR ( 'NONE', #12147, 1000.000000000000000 ) ;
#4209=CARTESIAN_POINT ( 'NONE',  ( 62.49999999999998579, 5.000000000000018652, -5.000000000000000000 ) ) ;
#4222=DIRECTION ( 'NONE',  ( 1.000000000000000000, 0.000000000000000000, 0.000000000000000000 ) ) ;
#4234=DIRECTION ( 'NONE',  ( 0.000000000000000000, 0.000000000000000000, -1.000000000000000000 ) ) ;
#4239=AXIS2_PLACEMENT_3D ( 'NONE', #11916, #12942, #3486 ) ;
#4244=CIRCLE ( 'NONE', #7993, 12.49999999999999645 ) ;
#4261=CARTESIAN_POINT ( 'NONE',  ( -62.49999999999997158, 32.50000000000001421, 15.00000000000000000 ) ) ;
#4269=DIRECTION ( 'NONE',  ( 1.000000000000000000, -0.000000000000000000, 0.000000000000000000 ) ) ;
#4272=AXIS2_PLACEMENT_3D ( 'NONE', #10918, #2764, #10848 ) ;
#4275=CARTESIAN_POINT ( 'NONE',  ( -74.99999999999997158, 20.00000000000001421, 15.00000000000000000 ) ) ;
#4307=FACE_OUTER_BOUND ( 'NONE', #10089, .T. ) ;
#4308=CARTESIAN_POINT ( 'NONE',  ( -62.49999999999997158, 45.00000000000001421, 15.00000000000000000 ) ) ;
#4309=LINE ( 'NONE', #12046, #5826 ) ;
#4327=CARTESIAN_POINT ( 'NONE',  ( 2.649999999999988365, 15.00000000000001599, -9.999999999999998224 ) ) ;
#4355=CARTESIAN_POINT ( 'NONE',  ( 2.649999999999988365, 15.00000000000001599, 15.00000000000000000 ) ) ;
#4368=LINE ( 'NONE', #3610, #3931 ) ;
#4375=VECTOR ( 'NONE', #5966, 1000.000000000000000 ) ;
#4382=ORIENTED_EDGE ( 'NONE', *, *, #4677, .F. ) ;
#4403=DIRECTION ( 'NONE',  ( 0.000000000000000000, 1.000000000000000000, 0.000000000000000000 ) ) ;
#4404=EDGE_CURVE ( 'NONE', #408, #7877, #2229, .T. ) ;
#4437=FACE_BOUND ( 'NONE', #5334, .T. ) ;
#4452=CIRCLE ( 'NONE', #10198, 9.999999999999998224 ) ;
#4461=DIRECTION ( 'NONE',  ( -0.000000000000000000, -0.000000000000000000, 1.000000000000000000 ) ) ;
#4469=ADVANCED_FACE ( 'NONE', ( #4822 ), #10209, .T. ) ;
#4483=VECTOR ( 'NONE', #6192, 1000.000000000000000 ) ;
#4486=ORIENTED_EDGE ( 'NONE', *, *, #5120, .T. ) ;
#4498=ADVANCED_FACE ( 'NONE', ( #10137 ), #2815, .F. ) ;
#4500=EDGE_CURVE ( 'NONE', #2907, #178, #2671, .T. ) ;
#4504=CARTESIAN_POINT ( 'NONE',  ( 62.49999999999998579, 40.00000000000001421, 5.000000000000000000 ) ) ;
#4505=DIRECTION ( 'NONE',  ( -1.000000000000000000, 0.000000000000000000, 0.000000000000000000 ) ) ;
#4508=DIRECTION ( 'NONE',  ( 1.000000000000000000, 0.000000000000000000, 0.000000000000000000 ) ) ;
#4519=VECTOR ( 'NONE', #11952, 1000.000000000000000 ) ;
#4520=ORIENTED_EDGE ( 'NONE', *, *, #10942, .T. ) ;
#4538=VERTEX_POINT ( 'NONE', #3917 ) ;
#4540=EDGE_CURVE ( 'NONE', #10018, #7328, #6900, .T. ) ;
#4546=CYLINDRICAL_SURFACE ( 'NONE', #3803, 9.999999999999998224 ) ;
#4561=VECTOR ( 'NONE', #749, 1000.000000000000000 ) ;
#4573=VERTEX_POINT ( 'NONE', #8143 ) ;
#4575=DIRECTION ( 'NONE',  ( -0.000000000000000000, 0.000000000000000000, -1.000000000000000000 ) ) ;
#4577=DIRECTION ( 'NONE',  ( 0.000000000000000000, 0.000000000000000000, -1.000000000000000000 ) ) ;
#4582=EDGE_CURVE ( 'NONE', #11747, #13619, #2599, .T. ) ;
#4598=EDGE_CURVE ( 'NONE', #7759, #3701, #11804, .T. ) ;
#4599=EDGE_CURVE ( 'NONE', #13259, #11359, #13168, .T. ) ;
#4649=DIRECTION ( 'NONE',  ( -0.000000000000000000, -0.000000000000000000, 1.000000000000000000 ) ) ;
#4656=CIRCLE ( 'NONE', #5770, 2.649999999999987477 ) ;
#4661=CARTESIAN_POINT ( 'NONE',  ( -62.49999999999997158, 40.00000000000001421, 9.999999999999998224 ) ) ;
#4677=EDGE_CURVE ( 'NONE', #5173, #10123, #3418, .T. ) ;
#4678=CARTESIAN_POINT ( 'NONE',  ( 0.000000000000000000, 0.000000000000000000, 15.00000000000000000 ) ) ;
#4706=EDGE_CURVE ( 'NONE', #408, #9920, #10919, .T. ) ;
#4728=ORIENTED_EDGE ( 'NONE', *, *, #5120, .F. ) ;
#4730=AXIS2_PLACEMENT_3D ( 'NONE', #6820, #1614, #2592 ) ;
#4757=DIRECTION ( 'NONE',  ( 1.000000000000000000, -0.000000000000000000, 0.000000000000000000 ) ) ;
#4768=DIRECTION ( 'NONE',  ( -0.000000000000000000, -0.000000000000000000, 1.000000000000000000 ) ) ;
#4781=VERTEX_POINT ( 'NONE', #8214 ) ;
#4785=LINE ( 'NONE', #6111, #10430 ) ;
#4786=DIRECTION ( 'NONE',  ( 1.000000000000000000, 0.000000000000000000, 0.000000000000000000 ) ) ;
#4793=DIRECTION ( 'NONE',  ( -1.000000000000000000, 0.000000000000000000, 0.000000000000000000 ) ) ;
#4811=EDGE_CURVE ( 'NONE', #3296, #6833, #834, .T. ) ;
#4814=FACE_BOUND ( 'NONE', #9026, .T. ) ;
#4819=EDGE_CURVE ( 'NONE', #10123, #5173, #9333, .T. ) ;
#4822=FACE_OUTER_BOUND ( 'NONE', #4958, .T. ) ;
#4834=EDGE_CURVE ( 'NONE', #9183, #10142, #12329, .T. ) ;
#4856=DIRECTION ( 'NONE',  ( 0.000000000000000000, 1.000000000000000000, 0.000000000000000000 ) ) ;
#4871=DIRECTION ( 'NONE',  ( -0.000000000000000000, -0.000000000000000000, 1.000000000000000000 ) ) ;
#4878=VECTOR ( 'NONE', #4508, 1000.000000000000000 ) ;
#4899=EDGE_CURVE ( 'NONE', #6144, #11844, #8124, .T. ) ;
#4901=EDGE_CURVE ( 'NONE', #967, #10505, #2863, .T. ) ;
#4905=EDGE_LOOP ( 'NONE', ( #3549, #8860, #12221, #12290 ) ) ;
#4908=CIRCLE ( 'NONE', #11966, 2.649999999999985700 ) ;
#4910=DIRECTION ( 'NONE',  ( 1.000000000000000000, 0.000000000000000000, 0.000000000000000000 ) ) ;
#4943=ORIENTED_EDGE ( 'NONE', *, *, #12589, .T. ) ;
#4945=LINE ( 'NONE', #1668, #7768 ) ;
#4952=ADVANCED_FACE ( 'NONE', ( #1673 ), #10191, .F. ) ;
#4958=EDGE_LOOP ( 'NONE', ( #3252, #8711, #12908, #9791 ) ) ;
#4960=CARTESIAN_POINT ( 'NONE',  ( 75.00000000000000000, 32.50000000000001421, -9.999999999999998224 ) ) ;
#4968=DIRECTION ( 'NONE',  ( 1.000000000000000000, 0.000000000000000000, 0.000000000000000000 ) ) ;
#4981=AXIS2_PLACEMENT_3D ( 'NONE', #12216, #8077, #4968 ) ;
#4983=PLANE ( 'NONE',  #856 ) ;
#5017=EDGE_CURVE ( 'NONE', #10229, #4573, #10114, .T. ) ;
#5021=AXIS2_PLACEMENT_3D ( 'NONE', #1654, #5898, #10095 ) ;
#5023=DIRECTION ( 'NONE',  ( -0.000000000000000000, -0.000000000000000000, -1.000000000000000000 ) ) ;
#5045=DIRECTION ( 'NONE',  ( -0.000000000000000000, 0.000000000000000000, -1.000000000000000000 ) ) ;
#5047=DIRECTION ( 'NONE',  ( 0.000000000000000000, -1.000000000000000000, 0.000000000000000000 ) ) ;
#5064=DIRECTION ( 'NONE',  ( 0.000000000000000000, -0.000000000000000000, 1.000000000000000000 ) ) ;
#5097=ORIENTED_EDGE ( 'NONE', *, *, #11961, .T. ) ;
#5112=ORIENTED_EDGE ( 'NONE', *, *, #2212, .T. ) ;
#5120=EDGE_CURVE ( 'NONE', #10107, #6120, #4178, .T. ) ;
#5130=VERTEX_POINT ( 'NONE', #12800 ) ;
#5158=CARTESIAN_POINT ( 'NONE',  ( -2.649999999999987477, 15.00000000000001599, 15.00000000000000178 ) ) ;
#5173=VERTEX_POINT ( 'NONE', #8534 ) ;
#5181=DIRECTION ( 'NONE',  ( 1.000000000000000000, -0.000000000000000000, 0.000000000000000000 ) ) ;
#5195=EDGE_CURVE ( 'NONE', #10003, #9042, #4908, .T. ) ;
#5201=FACE_OUTER_BOUND ( 'NONE', #6375, .T. ) ;
#5206=AXIS2_PLACEMENT_3D ( 'NONE', #4198, #6152, #932 ) ;
#5242=VECTOR ( 'NONE', #1043, 1000.000000000000000 ) ;
#5246=CARTESIAN_POINT ( 'NONE',  ( 10.00000000000000000, 15.00000000000001776, 15.00000000000000000 ) ) ;
#5263=DIRECTION ( 'NONE',  ( 0.000000000000000000, 0.000000000000000000, -1.000000000000000000 ) ) ;
#5281=ORIENTED_EDGE ( 'NONE', *, *, #1272, .T. ) ;
#5291=VECTOR ( 'NONE', #6253, 1000.000000000000000 ) ;
#5296=CARTESIAN_POINT ( 'NONE',  ( -62.49999999999997158, 32.50000000000001421, -9.999999999999998224 ) ) ;
#5310=AXIS2_PLACEMENT_3D ( 'NONE', #12605, #10532, #1040 ) ;
#5334=EDGE_LOOP ( 'NONE', ( #3997, #9660 ) ) ;
#5356=CARTESIAN_POINT ( 'NONE',  ( 2.649999999999987477, 15.00000000000001599, 15.00000000000000178 ) ) ;
#5372=ORIENTED_EDGE ( 'NONE', *, *, #81, .F. ) ;
#5375=DIRECTION ( 'NONE',  ( 0.000000000000000000, -0.000000000000000000, 1.000000000000000000 ) ) ;
#5382=LINE ( 'NONE', #11600, #11884 ) ;
#5393=AXIS2_PLACEMENT_3D ( 'NONE', #9562, #85, #787 ) ;
#5418=AXIS2_PLACEMENT_3D ( 'NONE', #4209, #2967, #13660 ) ;
#5423=DIRECTION ( 'NONE',  ( 0.000000000000000000, -0.000000000000000000, 1.000000000000000000 ) ) ;
#5465=CARTESIAN_POINT ( 'NONE',  ( -62.49999999999997158, 32.50000000000001421, 15.00000000000000000 ) ) ;
#5482=MECHANICAL_DESIGN_GEOMETRIC_PRESENTATION_REPRESENTATION('',(#2828),#2373);
#5483=ORIENTED_EDGE ( 'NONE', *, *, #12589, .F. ) ;
#5486=DIRECTION ( 'NONE',  ( -0.000000000000000000, -0.000000000000000000, 1.000000000000000000 ) ) ;
#5489=CARTESIAN_POINT ( 'NONE',  ( -59.84999999999998721, 32.50000000000001421, 9.999999999999998224 ) ) ;
#5492=AXIS2_PLACEMENT_3D ( 'NONE', #4275, #4403, #8493 ) ;
#5500=ORIENTED_EDGE ( 'NONE', *, *, #9083, .F. ) ;
#5511=CARTESIAN_POINT ( 'NONE',  ( -65.14999999999996305, 32.50000000000001421, -9.999999999999998224 ) ) ;
#5528=ADVANCED_FACE ( 'NONE', ( #5201 ), #2707, .T. ) ;
#5550=( NAMED_UNIT ( * ) SI_UNIT ( $, .STERADIAN. ) SOLID_ANGLE_UNIT ( ) );
#5590=DIRECTION ( 'NONE',  ( 0.000000000000000000, 1.000000000000000000, 0.000000000000000000 ) ) ;
#5593=VECTOR ( 'NONE', #11208, 1000.000000000000000 ) ;
#5595=LINE ( 'NONE', #1279, #9504 ) ;
#5601=EDGE_LOOP ( 'NONE', ( #1734, #390, #9539, #311 ) ) ;
#5633=EDGE_LOOP ( 'NONE', ( #10769, #3055, #212, #10386, #5810, #5097, #11215, #7977, #12189, #6524 ) ) ;
#5636=ORIENTED_EDGE ( 'NONE', *, *, #587, .T. ) ;
#5663=ADVANCED_FACE ( 'NONE', ( #5937 ), #3312, .F. ) ;
#5770=AXIS2_PLACEMENT_3D ( 'NONE', #603, #7138, #4786 ) ;
#5788=CARTESIAN_POINT ( 'NONE',  ( -62.49999999999997158, 45.00000000000001421, -15.00000000000000000 ) ) ;
#5789=ORIENTED_EDGE ( 'NONE', *, *, #3217, .T. ) ;
#5795=CARTESIAN_POINT ( 'NONE',  ( -9.999999999999998224, 15.00000000000001776, 15.00000000000000000 ) ) ;
#5810=ORIENTED_EDGE ( 'NONE', *, *, #8070, .T. ) ;
#5819=FACE_OUTER_BOUND ( 'NONE', #9398, .T. ) ;
#5826=VECTOR ( 'NONE', #4649, 1000.000000000000000 ) ;
#5828=CARTESIAN_POINT ( 'NONE',  ( 0.000000000000000000, 0.000000000000000000, 0.000000000000000000 ) ) ;
#5829=DIRECTION ( 'NONE',  ( 0.000000000000000000, -0.000000000000000000, 1.000000000000000000 ) ) ;
#5859=VECTOR ( 'NONE', #11174, 1000.000000000000000 ) ;
#5860=EDGE_CURVE ( 'NONE', #11777, #7974, #11530, .T. ) ;
#5861=ORIENTED_EDGE ( 'NONE', *, *, #10696, .F. ) ;
#5865=DIRECTION ( 'NONE',  ( 0.000000000000000000, 0.000000000000000000, -1.000000000000000000 ) ) ;
#5885=FACE_BOUND ( 'NONE', #9509, .T. ) ;
#5886=EDGE_CURVE ( 'NONE', #6144, #967, #10481, .T. ) ;
#5895=CARTESIAN_POINT ( 'NONE',  ( 10.00000000000000000, 0.000000000000000000, -9.999999999999998224 ) ) ;
#5898=DIRECTION ( 'NONE',  ( -0.000000000000000000, -0.000000000000000000, 1.000000000000000000 ) ) ;
#5921=DIRECTION ( 'NONE',  ( 1.000000000000000000, 0.000000000000000000, 0.000000000000000000 ) ) ;
#5927=DIRECTION ( 'NONE',  ( 1.000000000000000000, 0.000000000000000000, 0.000000000000000000 ) ) ;
#5937=FACE_OUTER_BOUND ( 'NONE', #10317, .T. ) ;
#5947=CARTESIAN_POINT ( 'NONE',  ( -9.999999999999996447, 25.00000000000001776, 15.00000000000000000 ) ) ;
#5950=EDGE_CURVE ( 'NONE', #10229, #6754, #5382, .T. ) ;
#5966=DIRECTION ( 'NONE',  ( 0.000000000000000000, 1.000000000000000000, 0.000000000000000000 ) ) ;
#5967=LINE ( 'NONE', #13332, #8881 ) ;
#5970=EDGE_CURVE ( 'NONE', #11894, #12887, #7515, .T. ) ;
#5977=LINE ( 'NONE', #548, #5593 ) ;
#5981=CARTESIAN_POINT ( 'NONE',  ( 32.49999999999998579, 40.00000000000001421, 5.000000000000002665 ) ) ;
#5990=DIRECTION ( 'NONE',  ( -1.000000000000000000, 0.000000000000000000, 1.224646799147353207E-16 ) ) ;
#6015=ORIENTED_EDGE ( 'NONE', *, *, #7381, .T. ) ;
#6030=CARTESIAN_POINT ( 'NONE',  ( 62.49999999999998579, 45.00000000000001421, 9.999999999999998224 ) ) ;
#6041=CARTESIAN_POINT ( 'NONE',  ( 62.49999999999998579, 40.00000000000001421, 0.000000000000000000 ) ) ;
#6048=AXIS2_PLACEMENT_3D ( 'NONE', #2551, #9880, #9948 ) ;
#6110=SURFACE_STYLE_FILL_AREA ( #2699 ) ;
#6111=CARTESIAN_POINT ( 'NONE',  ( 62.49999999999998579, 5.000000000000018652, 5.000000000000000000 ) ) ;
#6120=VERTEX_POINT ( 'NONE', #5511 ) ;
#6123=PRODUCT_DEFINITION_CONTEXT ( 'detailed design', #10613, 'design' ) ;
#6125=DIRECTION ( 'NONE',  ( -1.000000000000000000, 0.000000000000000000, -0.000000000000000000 ) ) ;
#6134=DIRECTION ( 'NONE',  ( 0.000000000000000000, 1.000000000000000000, 0.000000000000000000 ) ) ;
#6142=LINE ( 'NONE', #8411, #2626 ) ;
#6144=VERTEX_POINT ( 'NONE', #11857 ) ;
#6152=DIRECTION ( 'NONE',  ( -0.000000000000000000, -0.000000000000000000, 1.000000000000000000 ) ) ;
#6160=ORIENTED_EDGE ( 'NONE', *, *, #1775, .F. ) ;
#6168=CARTESIAN_POINT ( 'NONE',  ( -9.999999999999996447, 25.00000000000001776, 15.00000000000000000 ) ) ;
#6171=EDGE_LOOP ( 'NONE', ( #6540, #4520, #10921, #12851 ) ) ;
#6172=ORIENTED_EDGE ( 'NONE', *, *, #9481, .T. ) ;
#6178=( LENGTH_UNIT ( ) NAMED_UNIT ( * ) SI_UNIT ( .MILLI., .METRE. ) );
#6186=CARTESIAN_POINT ( 'NONE',  ( 62.49999999999998579, 45.00000000000001421, 15.00000000000000000 ) ) ;
#6188=ORIENTED_EDGE ( 'NONE', *, *, #10320, .T. ) ;
#6192=DIRECTION ( 'NONE',  ( -0.000000000000000000, 0.000000000000000000, -1.000000000000000000 ) ) ;
#6208=VECTOR ( 'NONE', #7178, 1000.000000000000000 ) ;
#6253=DIRECTION ( 'NONE',  ( 0.000000000000000000, -1.000000000000000000, 0.000000000000000000 ) ) ;
#6255=CARTESIAN_POINT ( 'NONE',  ( -74.99999999999997158, 20.00000000000001421, 15.00000000000000000 ) ) ;
#6314=ORIENTED_EDGE ( 'NONE', *, *, #3153, .F. ) ;
#6325=EDGE_CURVE ( 'NONE', #3166, #3701, #2866, .T. ) ;
#6331=PLANE ( 'NONE',  #2710 ) ;
#6340=CARTESIAN_POINT ( 'NONE',  ( 1.925929944387235853E-31, 15.00000000000001599, 15.00000000000000000 ) ) ;
#6375=EDGE_LOOP ( 'NONE', ( #633, #3436, #199, #6314 ) ) ;
#6377=CARTESIAN_POINT ( 'NONE',  ( 62.50000000000000000, 20.00000000000001421, 9.999999999999998224 ) ) ;
#6381=CARTESIAN_POINT ( 'NONE',  ( 9.999999999999994671, 20.00000000000001421, 9.999999999999998224 ) ) ;
#6428=ORIENTED_EDGE ( 'NONE', *, *, #7806, .T. ) ;
#6438=AXIS2_PLACEMENT_3D ( 'NONE', #3047, #8513, #12649 ) ;
#6444=VECTOR ( 'NONE', #7174, 1000.000000000000000 ) ;
#6464=VECTOR ( 'NONE', #3740, 1000.000000000000000 ) ;
#6473=CARTESIAN_POINT ( 'NONE',  ( -62.49999999999997158, 45.00000000000001421, 15.00000000000000000 ) ) ;
#6474=EDGE_CURVE ( 'NONE', #9060, #4066, #13055, .T. ) ;
#6475=ORIENTED_EDGE ( 'NONE', *, *, #4899, .T. ) ;
#6489=EDGE_CURVE ( 'NONE', #9824, #1019, #1794, .T. ) ;
#6497=EDGE_LOOP ( 'NONE', ( #7756, #5483, #6623, #8978, #13377, #12821, #2731, #13203, #6583, #12753, #1471, #11164 ) ) ;
#6502=LINE ( 'NONE', #7528, #8056 ) ;
#6511=ORIENTED_EDGE ( 'NONE', *, *, #4819, .F. ) ;
#6524=ORIENTED_EDGE ( 'NONE', *, *, #9063, .T. ) ;
#6538=ORIENTED_EDGE ( 'NONE', *, *, #1272, .F. ) ;
#6539=DIRECTION ( 'NONE',  ( -1.000000000000000000, 0.000000000000000000, 0.000000000000000000 ) ) ;
#6540=ORIENTED_EDGE ( 'NONE', *, *, #6620, .T. ) ;
#6543=DIRECTION ( 'NONE',  ( -0.000000000000000000, -0.000000000000000000, 1.000000000000000000 ) ) ;
#6569=ADVANCED_FACE ( 'NONE', ( #12378 ), #9138, .T. ) ;
#6574=EDGE_CURVE ( 'NONE', #919, #11844, #5967, .T. ) ;
#6583=ORIENTED_EDGE ( 'NONE', *, *, #4202, .F. ) ;
#6610=EDGE_CURVE ( 'NONE', #245, #13024, #4785, .T. ) ;
#6611=LINE ( 'NONE', #304, #11537 ) ;
#6620=EDGE_CURVE ( 'NONE', #10838, #11193, #673, .T. ) ;
#6623=ORIENTED_EDGE ( 'NONE', *, *, #4706, .F. ) ;
#6634=DIRECTION ( 'NONE',  ( -1.000000000000000000, 0.000000000000000000, 0.000000000000000000 ) ) ;
#6648=CIRCLE ( 'NONE', #6438, 2.649999999999985700 ) ;
#6649=CARTESIAN_POINT ( 'NONE',  ( -62.49999999999997158, 20.00000000000001421, 15.00000000000000000 ) ) ;
#6656=ORIENTED_EDGE ( 'NONE', *, *, #11921, .F. ) ;
#6660=CARTESIAN_POINT ( 'NONE',  ( -62.49999999999997158, 20.00000000000001421, -9.999999999999998224 ) ) ;
#6687=DIRECTION ( 'NONE',  ( 1.000000000000000000, 0.000000000000000000, 0.000000000000000000 ) ) ;
#6688=ORIENTED_EDGE ( 'NONE', *, *, #10596, .T. ) ;
#6707=EDGE_LOOP ( 'NONE', ( #7341, #9359, #3014, #6788 ) ) ;
#6708=DIRECTION ( 'NONE',  ( 1.000000000000000000, -0.000000000000000000, 0.000000000000000000 ) ) ;
#6716=ADVANCED_FACE ( 'NONE', ( #12514 ), #2135, .F. ) ;
#6721=ORIENTED_EDGE ( 'NONE', *, *, #5950, .T. ) ;
#6733=DIRECTION ( 'NONE',  ( -0.000000000000000000, 1.000000000000000000, -0.000000000000000000 ) ) ;
#6754=VERTEX_POINT ( 'NONE', #319 ) ;
#6758=CARTESIAN_POINT ( 'NONE',  ( -9.999999999999998224, 15.00000000000001776, -15.00000000000000000 ) ) ;
#6772=CARTESIAN_POINT ( 'NONE',  ( -59.84999999999998721, 32.50000000000001421, 15.00000000000000000 ) ) ;
#6788=ORIENTED_EDGE ( 'NONE', *, *, #3685, .F. ) ;
#6789=ORIENTED_EDGE ( 'NONE', *, *, #6574, .F. ) ;
#6820=CARTESIAN_POINT ( 'NONE',  ( -62.49999999999997158, 32.50000000000001421, 9.999999999999998224 ) ) ;
#6827=DIRECTION ( 'NONE',  ( -0.000000000000000000, -0.000000000000000000, 1.000000000000000000 ) ) ;
#6833=VERTEX_POINT ( 'NONE', #6381 ) ;
#6838=CARTESIAN_POINT ( 'NONE',  ( 1.925929944387235853E-31, 15.00000000000001599, 15.00000000000000178 ) ) ;
#6855=ADVANCED_FACE ( 'NONE', ( #3441 ), #4546, .T. ) ;
#6856=DIRECTION ( 'NONE',  ( -0.000000000000000000, 0.000000000000000000, -1.000000000000000000 ) ) ;
#6867=ORIENTED_EDGE ( 'NONE', *, *, #1036, .T. ) ;
#6900=LINE ( 'NONE', #2745, #12899 ) ;
#6912=AXIS2_PLACEMENT_3D ( 'NONE', #11571, #4234, #6125 ) ;
#6926=DIRECTION ( 'NONE',  ( -1.000000000000000000, 0.000000000000000000, 0.000000000000000000 ) ) ;
#6931=DIRECTION ( 'NONE',  ( 0.000000000000000000, 0.000000000000000000, -1.000000000000000000 ) ) ;
#6936=ORIENTED_EDGE ( 'NONE', *, *, #6474, .F. ) ;
#6949=AXIS2_PLACEMENT_3D ( 'NONE', #2334, #10713, #1289 ) ;
#6958=ORIENTED_EDGE ( 'NONE', *, *, #10231, .F. ) ;
#6969=CARTESIAN_POINT ( 'NONE',  ( 2.649999999999988365, 15.00000000000001599, 9.999999999999998224 ) ) ;
#6971=DIRECTION ( 'NONE',  ( -0.000000000000000000, -0.000000000000000000, 1.000000000000000000 ) ) ;
#6975=EDGE_LOOP ( 'NONE', ( #12454, #6428, #13326, #13255 ) ) ;
#7005=ORIENTED_EDGE ( 'NONE', *, *, #2975, .F. ) ;
#7018=CARTESIAN_POINT ( 'NONE',  ( -62.49999999999997158, 45.00000000000001421, 15.00000000000000000 ) ) ;
#7039=ORIENTED_EDGE ( 'NONE', *, *, #4901, .T. ) ;
#7041=AXIS2_PLACEMENT_3D ( 'NONE', #13108, #13038, #8772 ) ;
#7044=CARTESIAN_POINT ( 'NONE',  ( -9.999999999999996447, 25.00000000000001776, 15.00000000000000000 ) ) ;
#7059=ORIENTED_EDGE ( 'NONE', *, *, #2638, .T. ) ;
#7062=( NAMED_UNIT ( * ) SI_UNIT ( $, .STERADIAN. ) SOLID_ANGLE_UNIT ( ) );
#7063=DIRECTION ( 'NONE',  ( -1.000000000000000000, 0.000000000000000000, 0.000000000000000000 ) ) ;
#7098=DIRECTION ( 'NONE',  ( 0.000000000000000000, 0.000000000000000000, -1.000000000000000000 ) ) ;
#7120=AXIS2_PLACEMENT_3D ( 'NONE', #13492, #559, #4042 ) ;
#7122=DIRECTION ( 'NONE',  ( -0.000000000000000000, 0.000000000000000000, -1.000000000000000000 ) ) ;
#7138=DIRECTION ( 'NONE',  ( -0.000000000000000000, -0.000000000000000000, 1.000000000000000000 ) ) ;
#7162=EDGE_CURVE ( 'NONE', #12202, #4538, #10891, .T. ) ;
#7174=DIRECTION ( 'NONE',  ( 0.000000000000000000, 0.000000000000000000, -1.000000000000000000 ) ) ;
#7178=DIRECTION ( 'NONE',  ( -0.000000000000000000, -0.000000000000000000, -1.000000000000000000 ) ) ;
#7186=VERTEX_POINT ( 'NONE', #380 ) ;
#7189=VECTOR ( 'NONE', #3452, 1000.000000000000000 ) ;
#7206=LINE ( 'NONE', #12375, #5291 ) ;
#7227=CARTESIAN_POINT ( 'NONE',  ( 75.00000000000000000, 32.50000000000001421, 9.999999999999998224 ) ) ;
#7232=DIRECTION ( 'NONE',  ( 1.000000000000000000, 0.000000000000000000, 0.000000000000000000 ) ) ;
#7233=DIRECTION ( 'NONE',  ( 0.000000000000000000, 0.000000000000000000, -1.000000000000000000 ) ) ;
#7242=ORIENTED_EDGE ( 'NONE', *, *, #9892, .F. ) ;
#7246=CARTESIAN_POINT ( 'NONE',  ( -9.999999999999998224, 15.00000000000001776, -9.999999999999998224 ) ) ;
#7298=CARTESIAN_POINT ( 'NONE',  ( -62.49999999999997158, 32.50000000000001421, -9.999999999999998224 ) ) ;
#7302=DIRECTION ( 'NONE',  ( -0.000000000000000000, -0.000000000000000000, 1.000000000000000000 ) ) ;
#7304=DIRECTION ( 'NONE',  ( -1.000000000000000000, 0.000000000000000000, 0.000000000000000000 ) ) ;
#7328=VERTEX_POINT ( 'NONE', #6758 ) ;
#7339=DIRECTION ( 'NONE',  ( 1.000000000000000000, 0.000000000000000000, 0.000000000000000000 ) ) ;
#7341=ORIENTED_EDGE ( 'NONE', *, *, #8111, .T. ) ;
#7362=PLANE ( 'NONE',  #6912 ) ;
#7368=CARTESIAN_POINT ( 'NONE',  ( 1.925929944387235853E-31, 15.00000000000001599, -15.00000000000000000 ) ) ;
#7371=CYLINDRICAL_SURFACE ( 'NONE', #10732, 2.649999999999988365 ) ;
#7381=EDGE_CURVE ( 'NONE', #7922, #11193, #12617, .T. ) ;
#7390=ORIENTED_EDGE ( 'NONE', *, *, #4582, .F. ) ;
#7392=EDGE_CURVE ( 'NONE', #12054, #9060, #1974, .T. ) ;
#7415=FACE_OUTER_BOUND ( 'NONE', #12372, .T. ) ;
#7416=CIRCLE ( 'NONE', #12697, 9.999999999999998224 ) ;
#7429=FACE_OUTER_BOUND ( 'NONE', #9065, .T. ) ;
#7430=DIRECTION ( 'NONE',  ( 0.000000000000000000, 1.000000000000000000, 0.000000000000000000 ) ) ;
#7439=CARTESIAN_POINT ( 'NONE',  ( 0.000000000000000000, 20.00000000000001421, 9.999999999999998224 ) ) ;
#7441=DIRECTION ( 'NONE',  ( 1.000000000000000000, 0.000000000000000000, 0.000000000000000000 ) ) ;
#7478=ADVANCED_FACE ( 'NONE', ( #9512 ), #9579, .F. ) ;
#7488=CARTESIAN_POINT ( 'NONE',  ( -9.999999999999994671, 20.00000000000001421, 15.00000000000000000 ) ) ;
#7489=PLANE ( 'NONE',  #13557 ) ;
#7490=PLANE ( 'NONE',  #2682 ) ;
#7505=CARTESIAN_POINT ( 'NONE',  ( 62.49999999999998579, 40.00000000000001421, 9.999999999999998224 ) ) ;
#7515=LINE ( 'NONE', #2111, #8159 ) ;
#7528=CARTESIAN_POINT ( 'NONE',  ( -62.49999999999997158, 45.00000000000001421, -9.999999999999998224 ) ) ;
#7554=ORIENTED_EDGE ( 'NONE', *, *, #4598, .T. ) ;
#7555=CARTESIAN_POINT ( 'NONE',  ( -74.99999999999997158, 20.00000000000001421, 15.00000000000000000 ) ) ;
#7560=CARTESIAN_POINT ( 'NONE',  ( -62.49999999999997158, 32.50000000000001421, 15.00000000000000000 ) ) ;
#7590=ORIENTED_EDGE ( 'NONE', *, *, #3625, .F. ) ;
#7647=ADVANCED_FACE ( 'NONE', ( #10875 ), #8748, .F. ) ;
#7667=ADVANCED_FACE ( 'NONE', ( #9293 ), #827, .T. ) ;
#7668=DIRECTION ( 'NONE',  ( -0.000000000000000000, 1.000000000000000000, -0.000000000000000000 ) ) ;
#7689=CARTESIAN_POINT ( 'NONE',  ( -9.999999999999994671, 20.00000000000001421, 9.999999999999998224 ) ) ;
#7705=ORIENTED_EDGE ( 'NONE', *, *, #8983, .F. ) ;
#7707=EDGE_CURVE ( 'NONE', #4538, #3296, #4452, .T. ) ;
#7716=DIRECTION ( 'NONE',  ( -0.000000000000000000, -0.000000000000000000, 1.000000000000000000 ) ) ;
#7722=CARTESIAN_POINT ( 'NONE',  ( 62.50000000000000000, 32.50000000000001421, 15.00000000000000000 ) ) ;
#7725=ORIENTED_EDGE ( 'NONE', *, *, #5860, .T. ) ;
#7731=CIRCLE ( 'NONE', #12133, 2.649999999999987477 ) ;
#7737=FACE_OUTER_BOUND ( 'NONE', #4905, .T. ) ;
#7747=CARTESIAN_POINT ( 'NONE',  ( -62.49999999999997158, 20.00000000000001421, -15.00000000000000000 ) ) ;
#7754=CARTESIAN_POINT ( 'NONE',  ( 62.49999999999998579, 0.000000000000000000, -9.999999999999998224 ) ) ;
#7756=ORIENTED_EDGE ( 'NONE', *, *, #4500, .F. ) ;
#7759=VERTEX_POINT ( 'NONE', #7227 ) ;
#7763=DIRECTION ( 'NONE',  ( -1.000000000000000000, 0.000000000000000000, 0.000000000000000000 ) ) ;
#7768=VECTOR ( 'NONE', #10041, 1000.000000000000000 ) ;
#7785=CARTESIAN_POINT ( 'NONE',  ( -59.84999999999998721, 32.50000000000001421, 15.00000000000000000 ) ) ;
#7806=EDGE_CURVE ( 'NONE', #6754, #7186, #4945, .T. ) ;
#7810=ORIENTED_EDGE ( 'NONE', *, *, #12682, .F. ) ;
#7814=DIRECTION ( 'NONE',  ( 1.000000000000000000, 0.000000000000000000, -0.000000000000000000 ) ) ;
#7833=CARTESIAN_POINT ( 'NONE',  ( -62.49999999999997158, 32.50000000000001421, 9.999999999999998224 ) ) ;
#7851=CIRCLE ( 'NONE', #3622, 12.49999999999999645 ) ;
#7857=CARTESIAN_POINT ( 'NONE',  ( -62.49999999999997158, 32.50000000000001421, 15.00000000000000178 ) ) ;
#7877=VERTEX_POINT ( 'NONE', #4308 ) ;
#7881=ORIENTED_EDGE ( 'NONE', *, *, #9481, .F. ) ;
#7892=ORIENTED_EDGE ( 'NONE', *, *, #8540, .T. ) ;
#7911=CARTESIAN_POINT ( 'NONE',  ( -2.649999999999988809, 15.00000000000001599, -15.00000000000000000 ) ) ;
#7921=CARTESIAN_POINT ( 'NONE',  ( -62.49999999999997158, 32.50000000000001421, 15.00000000000000000 ) ) ;
#7922=VERTEX_POINT ( 'NONE', #2219 ) ;
#7923=CIRCLE ( 'NONE', #10996, 12.49999999999999645 ) ;
#7933=CARTESIAN_POINT ( 'NONE',  ( 10.00000000000000000, 25.00000000000001776, -15.00000000000000000 ) ) ;
#7934=CARTESIAN_POINT ( 'NONE',  ( 0.000000000000000000, 40.00000000000001421, 9.999999999999998224 ) ) ;
#7939=ADVANCED_FACE ( 'NONE', ( #7429 ), #7490, .T. ) ;
#7956=ORIENTED_EDGE ( 'NONE', *, *, #4540, .T. ) ;
#7959=ORIENTED_EDGE ( 'NONE', *, *, #2973, .T. ) ;
#7974=VERTEX_POINT ( 'NONE', #5158 ) ;
#7977=ORIENTED_EDGE ( 'NONE', *, *, #8218, .F. ) ;
#7993=AXIS2_PLACEMENT_3D ( 'NONE', #13164, #2668, #2528 ) ;
#7994=VERTEX_POINT ( 'NONE', #3336 ) ;
#8030=CARTESIAN_POINT ( 'NONE',  ( 32.49999999999998579, 5.000000000000018652, -4.999999999999996447 ) ) ;
#8047=EDGE_CURVE ( 'NONE', #6120, #10476, #2459, .T. ) ;
#8056=VECTOR ( 'NONE', #5590, 1000.000000000000000 ) ;
#8057=CARTESIAN_POINT ( 'NONE',  ( 10.00000000000000000, 0.000000000000000000, 9.999999999999998224 ) ) ;
#8070=EDGE_CURVE ( 'NONE', #12476, #13619, #11767, .T. ) ;
#8071=CARTESIAN_POINT ( 'NONE',  ( 62.49999999999998579, 32.50000000000001421, -9.999999999999998224 ) ) ;
#8077=DIRECTION ( 'NONE',  ( -0.000000000000000000, -0.000000000000000000, 1.000000000000000000 ) ) ;
#8085=EDGE_LOOP ( 'NONE', ( #9425, #9641, #247, #11110 ) ) ;
#8099=EDGE_LOOP ( 'NONE', ( #3481, #11092, #3604, #6867 ) ) ;
#8103=LINE ( 'NONE', #6041, #12969 ) ;
#8111=EDGE_CURVE ( 'NONE', #10142, #178, #1376, .T. ) ;
#8124=LINE ( 'NONE', #12468, #13501 ) ;
#8143=CARTESIAN_POINT ( 'NONE',  ( -62.49999999999997158, 20.00000000000001421, -15.00000000000000000 ) ) ;
#8152=DIRECTION ( 'NONE',  ( 1.000000000000000000, 0.000000000000000000, -0.000000000000000000 ) ) ;
#8158=CARTESIAN_POINT ( 'NONE',  ( 62.49999999999998579, 45.00000000000001421, 0.000000000000000000 ) ) ;
#8159=VECTOR ( 'NONE', #4269, 1000.000000000000000 ) ;
#8164=DIRECTION ( 'NONE',  ( 0.000000000000000000, -1.000000000000000000, 0.000000000000000000 ) ) ;
#8169=ORIENTED_EDGE ( 'NONE', *, *, #6474, .T. ) ;
#8171=LINE ( 'NONE', #5895, #4375 ) ;
#8175=CARTESIAN_POINT ( 'NONE',  ( 62.49999999999998579, 45.00000000000001421, 5.000000000000000000 ) ) ;
#8185=EDGE_LOOP ( 'NONE', ( #7005, #7554, #1155, #234 ) ) ;
#8187=ORIENTED_EDGE ( 'NONE', *, *, #4599, .F. ) ;
#8214=CARTESIAN_POINT ( 'NONE',  ( 10.00000000000000000, 15.00000000000001776, -9.999999999999998224 ) ) ;
#8218=EDGE_CURVE ( 'NONE', #7877, #3166, #13135, .T. ) ;
#8222=CARTESIAN_POINT ( 'NONE',  ( 62.49999999999998579, 45.00000000000001421, 15.00000000000000000 ) ) ;
#8230=EDGE_CURVE ( 'NONE', #9042, #10003, #3548, .T. ) ;
#8236=CARTESIAN_POINT ( 'NONE',  ( -62.49999999999997158, 40.00000000000001421, 0.000000000000000000 ) ) ;
#8266=CARTESIAN_POINT ( 'NONE',  ( -74.99999999999997158, 20.00000000000001421, 15.00000000000000000 ) ) ;
#8307=EDGE_CURVE ( 'NONE', #7974, #1019, #4656, .T. ) ;
#8329=FACE_BOUND ( 'NONE', #740, .T. ) ;
#8333=SHAPE_DEFINITION_REPRESENTATION ( #4125, #3897 ) ;
#8347=EDGE_LOOP ( 'NONE', ( #5372, #6475, #6789, #489, #12527, #8187, #10783, #1737 ) ) ;
#8359=ORIENTED_EDGE ( 'NONE', *, *, #9581, .F. ) ;
#8391=DIRECTION ( 'NONE',  ( -1.000000000000000000, 0.000000000000000000, 0.000000000000000000 ) ) ;
#8402=CARTESIAN_POINT ( 'NONE',  ( -65.14999999999996305, 32.50000000000001421, 15.00000000000000000 ) ) ;
#8409=ADVANCED_FACE ( 'NONE', ( #2628 ), #2701, .T. ) ;
#8411=CARTESIAN_POINT ( 'NONE',  ( -74.99999999999997158, 20.00000000000001421, -15.00000000000000000 ) ) ;
#8416=( GEOMETRIC_REPRESENTATION_CONTEXT ( 3 ) GLOBAL_UNCERTAINTY_ASSIGNED_CONTEXT ( ( #3435 ) ) GLOBAL_UNIT_ASSIGNED_CONTEXT ( ( #886, #2910, #7062 ) ) REPRESENTATION_CONTEXT ( 'NONE', 'WORKASPACE' ) );
#8453=ORIENTED_EDGE ( 'NONE', *, *, #3454, .T. ) ;
#8455=FACE_OUTER_BOUND ( 'NONE', #11248, .T. ) ;
#8474=DIRECTION ( 'NONE',  ( -0.000000000000000000, -0.000000000000000000, 1.000000000000000000 ) ) ;
#8493=DIRECTION ( 'NONE',  ( 0.000000000000000000, -0.000000000000000000, 1.000000000000000000 ) ) ;
#8509=ADVANCED_FACE ( 'NONE', ( #7415 ), #9474, .F. ) ;
#8511=EDGE_CURVE ( 'NONE', #4066, #12594, #1024, .T. ) ;
#8513=DIRECTION ( 'NONE',  ( -0.000000000000000000, -0.000000000000000000, 1.000000000000000000 ) ) ;
#8519=CARTESIAN_POINT ( 'NONE',  ( 10.00000000000000000, 15.00000000000001776, 9.999999999999998224 ) ) ;
#8522=ORIENTED_EDGE ( 'NONE', *, *, #10484, .T. ) ;
#8524=FACE_OUTER_BOUND ( 'NONE', #12696, .T. ) ;
#8534=CARTESIAN_POINT ( 'NONE',  ( -2.649999999999988365, 15.00000000000001599, -9.999999999999998224 ) ) ;
#8540=EDGE_CURVE ( 'NONE', #1320, #10107, #6648, .T. ) ;
#8542=CARTESIAN_POINT ( 'NONE',  ( -62.49999999999997158, 32.50000000000001421, -9.999999999999998224 ) ) ;
#8585=ORIENTED_EDGE ( 'NONE', *, *, #1775, .T. ) ;
#8590=DIRECTION ( 'NONE',  ( 0.000000000000000000, 0.000000000000000000, -1.000000000000000000 ) ) ;
#8594=DIRECTION ( 'NONE',  ( -0.000000000000000000, -0.000000000000000000, 1.000000000000000000 ) ) ;
#8662=CARTESIAN_POINT ( 'NONE',  ( -59.84999999999998721, 32.50000000000001421, 15.00000000000000178 ) ) ;
#8663=CARTESIAN_POINT ( 'NONE',  ( 0.000000000000000000, 0.000000000000000000, -15.00000000000000000 ) ) ;
#8669=CARTESIAN_POINT ( 'NONE',  ( 9.999999999999994671, 20.00000000000001421, -9.999999999999998224 ) ) ;
#8693=UNCERTAINTY_MEASURE_WITH_UNIT (LENGTH_MEASURE( 1.000000000000000082E-05 ), #6178, 'distance_accuracy_value', 'NONE');
#8694=ORIENTED_EDGE ( 'NONE', *, *, #2641, .F. ) ;
#8711=ORIENTED_EDGE ( 'NONE', *, *, #3153, .T. ) ;
#8732=FACE_OUTER_BOUND ( 'NONE', #8099, .T. ) ;
#8748=PLANE ( 'NONE',  #4239 ) ;
#8752=CARTESIAN_POINT ( 'NONE',  ( -62.49999999999997158, 32.50000000000001421, 15.00000000000000000 ) ) ;
#8770=CARTESIAN_POINT ( 'NONE',  ( 10.00000000000000000, 15.00000000000001776, -15.00000000000000000 ) ) ;
#8772=DIRECTION ( 'NONE',  ( 0.000000000000000000, -0.000000000000000000, 1.000000000000000000 ) ) ;
#8787=VERTEX_POINT ( 'NONE', #9875 ) ;
#8788=ORIENTED_EDGE ( 'NONE', *, *, #4899, .F. ) ;
#8792=LINE ( 'NONE', #3469, #9782 ) ;
#8801=LINE ( 'NONE', #2501, #2706 ) ;
#8812=EDGE_CURVE ( 'NONE', #1019, #7974, #7731, .T. ) ;
#8818=CYLINDRICAL_SURFACE ( 'NONE', #11304, 2.649999999999985700 ) ;
#8848=ORIENTED_EDGE ( 'NONE', *, *, #4582, .T. ) ;
#8860=ORIENTED_EDGE ( 'NONE', *, *, #4706, .T. ) ;
#8880=ORIENTED_EDGE ( 'NONE', *, *, #5195, .F. ) ;
#8881=VECTOR ( 'NONE', #13194, 1000.000000000000000 ) ;
#8910=DIRECTION ( 'NONE',  ( -0.000000000000000000, -0.000000000000000000, -1.000000000000000000 ) ) ;
#8919=PLANE ( 'NONE',  #10260 ) ;
#8928=ADVANCED_FACE ( 'NONE', ( #10222 ), #4983, .T. ) ;
#8960=UNCERTAINTY_MEASURE_WITH_UNIT (LENGTH_MEASURE( 1.000000000000000082E-05 ), #2560, 'distance_accuracy_value', 'NONE');
#8970=DIRECTION ( 'NONE',  ( -1.000000000000000000, 0.000000000000000000, 0.000000000000000000 ) ) ;
#8977=LINE ( 'NONE', #11950, #1052 ) ;
#8978=ORIENTED_EDGE ( 'NONE', *, *, #3454, .F. ) ;
#8983=EDGE_CURVE ( 'NONE', #11359, #3701, #945, .T. ) ;
#8993=ORIENTED_EDGE ( 'NONE', *, *, #13414, .F. ) ;
#8996=DIRECTION ( 'NONE',  ( -0.000000000000000000, 1.000000000000000000, -0.000000000000000000 ) ) ;
#9026=EDGE_LOOP ( 'NONE', ( #389, #474 ) ) ;
#9042=VERTEX_POINT ( 'NONE', #5489 ) ;
#9043=VERTEX_POINT ( 'NONE', #12536 ) ;
#9046=ORIENTED_EDGE ( 'NONE', *, *, #4811, .T. ) ;
#9047=EDGE_CURVE ( 'NONE', #13190, #345, #11254, .T. ) ;
#9048=FACE_OUTER_BOUND ( 'NONE', #6707, .T. ) ;
#9060=VERTEX_POINT ( 'NONE', #2222 ) ;
#9062=ORIENTED_EDGE ( 'NONE', *, *, #3625, .T. ) ;
#9063=EDGE_CURVE ( 'NONE', #1386, #9183, #1976, .T. ) ;
#9065=EDGE_LOOP ( 'NONE', ( #313, #6958, #7705, #6188 ) ) ;
#9083=EDGE_CURVE ( 'NONE', #11777, #9824, #9490, .T. ) ;
#9106=FACE_OUTER_BOUND ( 'NONE', #11380, .T. ) ;
#9107=AXIS2_PLACEMENT_3D ( 'NONE', #11201, #13264, #7063 ) ;
#9119=VERTEX_POINT ( 'NONE', #8669 ) ;
#9137=SURFACE_SIDE_STYLE ('',( #6110 ) ) ;
#9138=CYLINDRICAL_SURFACE ( 'NONE', #262, 12.49999999999999645 ) ;
#9155=AXIS2_PLACEMENT_3D ( 'NONE', #7857, #776, #11230 ) ;
#9169=ORIENTED_EDGE ( 'NONE', *, *, #6325, .T. ) ;
#9175=AXIS2_PLACEMENT_3D ( 'NONE', #13298, #7098, #3842 ) ;
#9180=DIRECTION ( 'NONE',  ( -1.224646799147353207E-16, 0.000000000000000000, -1.000000000000000000 ) ) ;
#9183=VERTEX_POINT ( 'NONE', #6649 ) ;
#9185=ORIENTED_EDGE ( 'NONE', *, *, #2544, .F. ) ;
#9211=CARTESIAN_POINT ( 'NONE',  ( -59.84999999999998721, 32.50000000000001421, -15.00000000000000000 ) ) ;
#9221=VERTEX_POINT ( 'NONE', #1363 ) ;
#9255=EDGE_LOOP ( 'NONE', ( #9593, #4486, #8694, #2642 ) ) ;
#9258=DIRECTION ( 'NONE',  ( -1.000000000000000000, 0.000000000000000000, 1.224646799147353207E-16 ) ) ;
#9260=PLANE ( 'NONE',  #5418 ) ;
#9275=FILL_AREA_STYLE_COLOUR ( '', #10385 ) ;
#9286=ORIENTED_EDGE ( 'NONE', *, *, #8070, .F. ) ;
#9290=LINE ( 'NONE', #13, #4483 ) ;
#9293=FACE_OUTER_BOUND ( 'NONE', #9759, .T. ) ;
#9297=AXIS2_PLACEMENT_3D ( 'NONE', #6255, #12714, #888 ) ;
#9298=CARTESIAN_POINT ( 'NONE',  ( 62.49999999999998579, 45.00000000000001421, -5.000000000000000000 ) ) ;
#9327=ORIENTED_EDGE ( 'NONE', *, *, #2720, .F. ) ;
#9329=ORIENTED_EDGE ( 'NONE', *, *, #3984, .F. ) ;
#9333=CIRCLE ( 'NONE', #2693, 2.649999999999988365 ) ;
#9341=ORIENTED_EDGE ( 'NONE', *, *, #7707, .T. ) ;
#9359=ORIENTED_EDGE ( 'NONE', *, *, #590, .T. ) ;
#9360=ORIENTED_EDGE ( 'NONE', *, *, #10318, .F. ) ;
#9369=FACE_OUTER_BOUND ( 'NONE', #13294, .T. ) ;
#9373=LINE ( 'NONE', #7439, #9812 ) ;
#9398=EDGE_LOOP ( 'NONE', ( #2399, #12773, #9757, #4382 ) ) ;
#9425=ORIENTED_EDGE ( 'NONE', *, *, #8230, .T. ) ;
#9433=CARTESIAN_POINT ( 'NONE',  ( -74.99999999999997158, 32.50000000000001421, 15.00000000000000000 ) ) ;
#9456=CARTESIAN_POINT ( 'NONE',  ( 32.49999999999998579, 45.00000000000001421, 5.000000000000003553 ) ) ;
#9474=PLANE ( 'NONE',  #9297 ) ;
#9481=EDGE_CURVE ( 'NONE', #12594, #10838, #2005, .T. ) ;
#9490=CIRCLE ( 'NONE', #5310, 2.649999999999988365 ) ;
#9498=LINE ( 'NONE', #9433, #3453 ) ;
#9504=VECTOR ( 'NONE', #7668, 1000.000000000000000 ) ;
#9509=EDGE_LOOP ( 'NONE', ( #11407, #13094 ) ) ;
#9511=LINE ( 'NONE', #12809, #13132 ) ;
#9512=FACE_OUTER_BOUND ( 'NONE', #2538, .T. ) ;
#9538=EDGE_LOOP ( 'NONE', ( #10803, #1356 ) ) ;
#9539=ORIENTED_EDGE ( 'NONE', *, *, #6489, .T. ) ;
#9562=CARTESIAN_POINT ( 'NONE',  ( -62.49999999999997158, 45.00000000000001421, 0.000000000000000000 ) ) ;
#9570=AXIS2_PLACEMENT_3D ( 'NONE', #7560, #2564, #10992 ) ;
#9575=CARTESIAN_POINT ( 'NONE',  ( -62.49999999999997158, 32.50000000000001421, -15.00000000000000000 ) ) ;
#9579=CYLINDRICAL_SURFACE ( 'NONE', #2450, 2.649999999999985700 ) ;
#9581=EDGE_CURVE ( 'NONE', #5130, #12476, #5595, .T. ) ;
#9593=ORIENTED_EDGE ( 'NONE', *, *, #343, .F. ) ;
#9621=VERTEX_POINT ( 'NONE', #8770 ) ;
#9631=CARTESIAN_POINT ( 'NONE',  ( -62.49999999999997158, 32.50000000000001421, 15.00000000000000000 ) ) ;
#9634=CARTESIAN_POINT ( 'NONE',  ( -62.49999999999997158, 32.50000000000001421, 9.999999999999998224 ) ) ;
#9641=ORIENTED_EDGE ( 'NONE', *, *, #267, .T. ) ;
#9657=ADVANCED_FACE ( 'NONE', ( #7737 ), #9739, .T. ) ;
#9660=ORIENTED_EDGE ( 'NONE', *, *, #9047, .T. ) ;
#9674=ORIENTED_EDGE ( 'NONE', *, *, #8230, .F. ) ;
#9689=ORIENTED_EDGE ( 'NONE', *, *, #7806, .F. ) ;
#9691=( NAMED_UNIT ( * ) PLANE_ANGLE_UNIT ( ) SI_UNIT ( $, .RADIAN. ) );
#9700=CIRCLE ( 'NONE', #3737, 12.49999999999999645 ) ;
#9711=CARTESIAN_POINT ( 'NONE',  ( 62.49999999999998579, 45.00000000000001421, 5.000000000000000000 ) ) ;
#9739=CYLINDRICAL_SURFACE ( 'NONE', #2197, 12.49999999999999645 ) ;
#9755=AXIS2_PLACEMENT_3D ( 'NONE', #2718, #13209, #2931 ) ;
#9757=ORIENTED_EDGE ( 'NONE', *, *, #11921, .T. ) ;
#9759=EDGE_LOOP ( 'NONE', ( #7059, #4943, #12289, #10090 ) ) ;
#9763=DIRECTION ( 'NONE',  ( -0.000000000000000000, 0.000000000000000000, -1.000000000000000000 ) ) ;
#9774=ORIENTED_EDGE ( 'NONE', *, *, #2973, .F. ) ;
#9782=VECTOR ( 'NONE', #409, 1000.000000000000000 ) ;
#9791=ORIENTED_EDGE ( 'NONE', *, *, #6610, .F. ) ;
#9812=VECTOR ( 'NONE', #3972, 1000.000000000000000 ) ;
#9824=VERTEX_POINT ( 'NONE', #6969 ) ;
#9840=ORIENTED_EDGE ( 'NONE', *, *, #13414, .T. ) ;
#9849=AXIS2_PLACEMENT_3D ( 'NONE', #9575, #8474, #7441 ) ;
#9861=LINE ( 'NONE', #1475, #12013 ) ;
#9875=CARTESIAN_POINT ( 'NONE',  ( 9.999999999999994671, 20.00000000000001421, -15.00000000000000000 ) ) ;
#9880=DIRECTION ( 'NONE',  ( -0.000000000000000000, -0.000000000000000000, 1.000000000000000000 ) ) ;
#9892=EDGE_CURVE ( 'NONE', #9621, #8787, #3709, .T. ) ;
#9920=VERTEX_POINT ( 'NONE', #3089 ) ;
#9921=DIRECTION ( 'NONE',  ( -1.000000000000000000, 0.000000000000000000, -0.000000000000000000 ) ) ;
#9923=EDGE_CURVE ( 'NONE', #13190, #5173, #12793, .T. ) ;
#9935=VECTOR ( 'NONE', #5486, 1000.000000000000000 ) ;
#9948=DIRECTION ( 'NONE',  ( 1.000000000000000000, 0.000000000000000000, 0.000000000000000000 ) ) ;
#9973=VECTOR ( 'NONE', #12668, 1000.000000000000000 ) ;
#9982=LINE ( 'NONE', #7018, #2520 ) ;
#9989=EDGE_CURVE ( 'NONE', #5130, #3296, #12416, .T. ) ;
#10003=VERTEX_POINT ( 'NONE', #3986 ) ;
#10018=VERTEX_POINT ( 'NONE', #7246 ) ;
#10026=DIRECTION ( 'NONE',  ( 1.000000000000000000, 0.000000000000000000, 0.000000000000000000 ) ) ;
#10028=LINE ( 'NONE', #8175, #10959 ) ;
#10041=DIRECTION ( 'NONE',  ( -0.000000000000000000, 0.000000000000000000, -1.000000000000000000 ) ) ;
#10077=DIRECTION ( 'NONE',  ( -0.000000000000000000, -0.000000000000000000, 1.000000000000000000 ) ) ;
#10085=PLANE ( 'NONE',  #4272 ) ;
#10089=EDGE_LOOP ( 'NONE', ( #13555, #7242, #7590, #3938, #6538, #11538, #8169, #3808, #6172, #164 ) ) ;
#10090=ORIENTED_EDGE ( 'NONE', *, *, #9063, .F. ) ;
#10095=DIRECTION ( 'NONE',  ( -1.000000000000000000, 0.000000000000000000, 0.000000000000000000 ) ) ;
#10105=ORIENTED_EDGE ( 'NONE', *, *, #8218, .T. ) ;
#10107=VERTEX_POINT ( 'NONE', #1127 ) ;
#10114=LINE ( 'NONE', #624, #1136 ) ;
#10123=VERTEX_POINT ( 'NONE', #4327 ) ;
#10137=FACE_OUTER_BOUND ( 'NONE', #5601, .T. ) ;
#10142=VERTEX_POINT ( 'NONE', #7488 ) ;
#10146=AXIS2_PLACEMENT_3D ( 'NONE', #7368, #8594, #3272 ) ;
#10167=( GEOMETRIC_REPRESENTATION_CONTEXT ( 3 ) GLOBAL_UNCERTAINTY_ASSIGNED_CONTEXT ( ( #8693 ) ) GLOBAL_UNIT_ASSIGNED_CONTEXT ( ( #6178, #2841, #2774 ) ) REPRESENTATION_CONTEXT ( 'NONE', 'WORKASPACE' ) );
#10186=CARTESIAN_POINT ( 'NONE',  ( 1.925929944387235853E-31, 15.00000000000001599, 9.999999999999998224 ) ) ;
#10191=CYLINDRICAL_SURFACE ( 'NONE', #7120, 2.649999999999988365 ) ;
#10198=AXIS2_PLACEMENT_3D ( 'NONE', #10186, #2999, #11427 ) ;
#10209=PLANE ( 'NONE',  #974 ) ;
#10222=FACE_OUTER_BOUND ( 'NONE', #3197, .T. ) ;
#10229=VERTEX_POINT ( 'NONE', #6660 ) ;
#10231=EDGE_CURVE ( 'NONE', #3701, #13024, #4368, .T. ) ;
#10233=DIRECTION ( 'NONE',  ( -0.000000000000000000, 0.000000000000000000, -1.000000000000000000 ) ) ;
#10236=LINE ( 'NONE', #1583, #4561 ) ;
#10244=ADVANCED_FACE ( 'NONE', ( #2493 ), #1443, .T. ) ;
#10251=MANIFOLD_SOLID_BREP ( 'M5 Clearance Hole1', #13084 ) ;
#10259=DIRECTION ( 'NONE',  ( 0.000000000000000000, 0.000000000000000000, -1.000000000000000000 ) ) ;
#10260=AXIS2_PLACEMENT_3D ( 'NONE', #5947, #7814, #13178 ) ;
#10263=CARTESIAN_POINT ( 'NONE',  ( 62.49999999999998579, 45.00000000000001421, 15.00000000000000000 ) ) ;
#10269=ORIENTED_EDGE ( 'NONE', *, *, #2257, .T. ) ;
#10283=EDGE_LOOP ( 'NONE', ( #6688, #441, #77, #3620, #4167, #8585, #9774, #3220, #6721, #3768, #9840, #8522 ) ) ;
#10288=LINE ( 'NONE', #727, #2984 ) ;
#10290=CARTESIAN_POINT ( 'NONE',  ( 62.49999999999998579, 45.00000000000001421, 9.999999999999998224 ) ) ;
#10299=VERTEX_POINT ( 'NONE', #8662 ) ;
#10317=EDGE_LOOP ( 'NONE', ( #1632, #632, #79, #11445 ) ) ;
#10318=EDGE_CURVE ( 'NONE', #11844, #10505, #3738, .T. ) ;
#10320=EDGE_CURVE ( 'NONE', #11359, #245, #8103, .T. ) ;
#10322=CARTESIAN_POINT ( 'NONE',  ( 1.925929944387235853E-31, 15.00000000000001599, -9.999999999999998224 ) ) ;
#10344=DIRECTION ( 'NONE',  ( 0.000000000000000000, -0.000000000000000000, 1.000000000000000000 ) ) ;
#10374=DIRECTION ( 'NONE',  ( -0.000000000000000000, -0.000000000000000000, 1.000000000000000000 ) ) ;
#10385=COLOUR_RGB ( '',0.8941176470588234615, 0.8941176470588234615, 0.8941176470588234615 ) ;
#10386=ORIENTED_EDGE ( 'NONE', *, *, #9581, .T. ) ;
#10393=DIRECTION ( 'NONE',  ( 1.000000000000000000, 0.000000000000000000, -0.000000000000000000 ) ) ;
#10430=VECTOR ( 'NONE', #8996, 1000.000000000000000 ) ;
#10438=DIRECTION ( 'NONE',  ( 0.000000000000000000, 0.000000000000000000, 1.000000000000000000 ) ) ;
#10459=DIRECTION ( 'NONE',  ( -1.000000000000000000, 0.000000000000000000, -0.000000000000000000 ) ) ;
#10460=CARTESIAN_POINT ( 'NONE',  ( 62.49999999999998579, 45.00000000000001421, 0.000000000000000000 ) ) ;
#10465=PRODUCT_DEFINITION ( 'UNKNOWN', '', #10800, #6123 ) ;
#10473=DIRECTION ( 'NONE',  ( 1.000000000000000000, 0.000000000000000000, 0.000000000000000000 ) ) ;
#10474=ORIENTED_EDGE ( 'NONE', *, *, #11961, .F. ) ;
#10476=VERTEX_POINT ( 'NONE', #1651 ) ;
#10481=LINE ( 'NONE', #1905, #12565 ) ;
#10484=EDGE_CURVE ( 'NONE', #4781, #9119, #8171, .T. ) ;
#10505=VERTEX_POINT ( 'NONE', #1579 ) ;
#10532=DIRECTION ( 'NONE',  ( 0.000000000000000000, 0.000000000000000000, -1.000000000000000000 ) ) ;
#10596=EDGE_CURVE ( 'NONE', #9119, #9043, #8977, .T. ) ;
#10597=CARTESIAN_POINT ( 'NONE',  ( 62.49999999999998579, 20.00000000000001421, 15.00000000000000000 ) ) ;
#10599=PLANE ( 'NONE',  #2413 ) ;
#10609=EDGE_LOOP ( 'NONE', ( #9185, #6160, #3253, #8453 ) ) ;
#10613=APPLICATION_CONTEXT ( 'automotive_design' ) ;
#10645=VECTOR ( 'NONE', #5064, 1000.000000000000000 ) ;
#10661=PLANE ( 'NONE',  #2053 ) ;
#10677=DIRECTION ( 'NONE',  ( -0.000000000000000000, -0.000000000000000000, 1.000000000000000000 ) ) ;
#10678=ORIENTED_EDGE ( 'NONE', *, *, #13522, .T. ) ;
#10689=FACE_OUTER_BOUND ( 'NONE', #8085, .T. ) ;
#10696=EDGE_CURVE ( 'NONE', #967, #7922, #12360, .T. ) ;
#10697=VERTEX_POINT ( 'NONE', #3998 ) ;
#10713=DIRECTION ( 'NONE',  ( -0.000000000000000000, -0.000000000000000000, 1.000000000000000000 ) ) ;
#10720=ORIENTED_EDGE ( 'NONE', *, *, #8047, .F. ) ;
#10726=CARTESIAN_POINT ( 'NONE',  ( -2.649999999999988365, 15.00000000000001599, 15.00000000000000000 ) ) ;
#10732=AXIS2_PLACEMENT_3D ( 'NONE', #6340, #12399, #11580 ) ;
#10739=LINE ( 'NONE', #165, #3084 ) ;
#10758=CARTESIAN_POINT ( 'NONE',  ( 75.00000000000000000, 32.50000000000001421, -15.00000000000000000 ) ) ;
#10767=VECTOR ( 'NONE', #12106, 1000.000000000000000 ) ;
#10769=ORIENTED_EDGE ( 'NONE', *, *, #4834, .T. ) ;
#10771=EDGE_LOOP ( 'NONE', ( #3042, #2873 ) ) ;
#10783=ORIENTED_EDGE ( 'NONE', *, *, #3692, .F. ) ;
#10790=AXIS2_PLACEMENT_3D ( 'NONE', #12439, #10374, #3114 ) ;
#10800=PRODUCT_DEFINITION_FORMATION_WITH_SPECIFIED_SOURCE ( 'ANY', '', #2235, .NOT_KNOWN. ) ;
#10803=ORIENTED_EDGE ( 'NONE', *, *, #2641, .T. ) ;
#10820=CARTESIAN_POINT ( 'NONE',  ( 62.50000000000000000, 32.50000000000001421, -9.999999999999998224 ) ) ;
#10826=DIRECTION ( 'NONE',  ( -0.000000000000000000, -0.000000000000000000, -1.000000000000000000 ) ) ;
#10832=ADVANCED_FACE ( 'NONE', ( #3923 ), #2823, .F. ) ;
#10838=VERTEX_POINT ( 'NONE', #10758 ) ;
#10840=LINE ( 'NONE', #7747, #4519 ) ;
#10848=DIRECTION ( 'NONE',  ( -1.000000000000000000, 0.000000000000000000, -0.000000000000000000 ) ) ;
#10854=VERTEX_POINT ( 'NONE', #9456 ) ;
#10858=CARTESIAN_POINT ( 'NONE',  ( 62.49999999999998579, 32.50000000000001421, 15.00000000000000000 ) ) ;
#10873=AXIS2_PLACEMENT_3D ( 'NONE', #2636, #1659, #4793 ) ;
#10875=FACE_OUTER_BOUND ( 'NONE', #3398, .T. ) ;
#10891=LINE ( 'NONE', #5795, #1335 ) ;
#10902=ORIENTED_EDGE ( 'NONE', *, *, #9923, .T. ) ;
#10907=ADVANCED_FACE ( 'NONE', ( #182 ), #53, .F. ) ;
#10918=CARTESIAN_POINT ( 'NONE',  ( 0.000000000000000000, 0.000000000000000000, -9.999999999999998224 ) ) ;
#10919=CIRCLE ( 'NONE', #5206, 12.49999999999999645 ) ;
#10921=ORIENTED_EDGE ( 'NONE', *, *, #1036, .F. ) ;
#10942=EDGE_CURVE ( 'NONE', #11193, #9043, #7923, .T. ) ;
#10959=VECTOR ( 'NONE', #675, 1000.000000000000000 ) ;
#10970=ADVANCED_FACE ( 'NONE', ( #3501, #4814, #13095 ), #2523, .F. ) ;
#10975=CARTESIAN_POINT ( 'NONE',  ( -74.99999999999997158, 32.50000000000001421, -9.999999999999998224 ) ) ;
#10990=DIRECTION ( 'NONE',  ( 0.000000000000000000, 0.000000000000000000, 1.000000000000000000 ) ) ;
#10992=DIRECTION ( 'NONE',  ( 1.000000000000000000, 0.000000000000000000, 0.000000000000000000 ) ) ;
#10996=AXIS2_PLACEMENT_3D ( 'NONE', #10820, #12139, #1337 ) ;
#11092=ORIENTED_EDGE ( 'NONE', *, *, #12945, .F. ) ;
#11093=CIRCLE ( 'NONE', #59, 2.649999999999985700 ) ;
#11102=VECTOR ( 'NONE', #11960, 1000.000000000000000 ) ;
#11110=ORIENTED_EDGE ( 'NONE', *, *, #12031, .F. ) ;
#11164=ORIENTED_EDGE ( 'NONE', *, *, #590, .F. ) ;
#11174=DIRECTION ( 'NONE',  ( 1.000000000000000000, -0.000000000000000000, 0.000000000000000000 ) ) ;
#11193=VERTEX_POINT ( 'NONE', #4960 ) ;
#11200=PRESENTATION_STYLE_ASSIGNMENT (( #1721 ) ) ;
#11201=CARTESIAN_POINT ( 'NONE',  ( -62.49999999999997158, 32.50000000000001421, -15.00000000000000000 ) ) ;
#11208=DIRECTION ( 'NONE',  ( 0.000000000000000000, -0.000000000000000000, 1.000000000000000000 ) ) ;
#11215=ORIENTED_EDGE ( 'NONE', *, *, #2081, .T. ) ;
#11230=DIRECTION ( 'NONE',  ( 1.000000000000000000, 0.000000000000000000, 0.000000000000000000 ) ) ;
#11248=EDGE_LOOP ( 'NONE', ( #2835, #9046, #5112, #8359 ) ) ;
#11253=DIRECTION ( 'NONE',  ( -0.000000000000000000, 0.000000000000000000, -1.000000000000000000 ) ) ;
#11254=CIRCLE ( 'NONE', #10146, 2.649999999999988809 ) ;
#11268=ORIENTED_EDGE ( 'NONE', *, *, #1200, .T. ) ;
#11291=AXIS2_PLACEMENT_3D ( 'NONE', #7298, #11507, #975 ) ;
#11304=AXIS2_PLACEMENT_3D ( 'NONE', #8752, #7716, #173 ) ;
#11359=VERTEX_POINT ( 'NONE', #7505 ) ;
#11363=VECTOR ( 'NONE', #10677, 1000.000000000000000 ) ;
#11371=DIRECTION ( 'NONE',  ( 0.000000000000000000, 0.000000000000000000, -1.000000000000000000 ) ) ;
#11380=EDGE_LOOP ( 'NONE', ( #665, #7959, #9329, #6936 ) ) ;
#11383=CIRCLE ( 'NONE', #9175, 12.49999999999999645 ) ;
#11407=ORIENTED_EDGE ( 'NONE', *, *, #4819, .T. ) ;
#11409=ORIENTED_EDGE ( 'NONE', *, *, #4404, .T. ) ;
#11418=DIRECTION ( 'NONE',  ( 1.000000000000000000, 0.000000000000000000, 0.000000000000000000 ) ) ;
#11427=DIRECTION ( 'NONE',  ( -1.000000000000000000, 0.000000000000000000, 0.000000000000000000 ) ) ;
#11445=ORIENTED_EDGE ( 'NONE', *, *, #4834, .F. ) ;
#11477=CARTESIAN_POINT ( 'NONE',  ( 1.925929944387235853E-31, 15.00000000000001599, -15.00000000000000000 ) ) ;
#11499=ORIENTED_EDGE ( 'NONE', *, *, #10231, .T. ) ;
#11507=DIRECTION ( 'NONE',  ( 0.000000000000000000, 0.000000000000000000, -1.000000000000000000 ) ) ;
#11509=DIRECTION ( 'NONE',  ( -1.000000000000000000, 0.000000000000000000, 0.000000000000000000 ) ) ;
#11529=DIRECTION ( 'NONE',  ( 1.000000000000000000, 0.000000000000000000, 0.000000000000000000 ) ) ;
#11530=LINE ( 'NONE', #13507, #833 ) ;
#11537=VECTOR ( 'NONE', #11721, 1000.000000000000000 ) ;
#11538=ORIENTED_EDGE ( 'NONE', *, *, #12746, .T. ) ;
#11558=AXIS2_PLACEMENT_3D ( 'NONE', #12923, #3536, #12994 ) ;
#11571=CARTESIAN_POINT ( 'NONE',  ( 0.000000000000000000, 0.000000000000000000, 9.999999999999998224 ) ) ;
#11580=DIRECTION ( 'NONE',  ( 1.000000000000000000, 0.000000000000000000, 0.000000000000000000 ) ) ;
#11600=CARTESIAN_POINT ( 'NONE',  ( 0.000000000000000000, 20.00000000000001421, -9.999999999999998224 ) ) ;
#11620=CIRCLE ( 'NONE', #9849, 2.649999999999985700 ) ;
#11630=AXIS2_PLACEMENT_3D ( 'NONE', #13266, #4856, #604 ) ;
#11674=ORIENTED_EDGE ( 'NONE', *, *, #12031, .T. ) ;
#11678=EDGE_CURVE ( 'NONE', #7186, #7328, #7206, .T. ) ;
#11711=CARTESIAN_POINT ( 'NONE',  ( -62.49999999999997158, 45.00000000000001421, -9.999999999999998224 ) ) ;
#11721=DIRECTION ( 'NONE',  ( 0.000000000000000000, -0.000000000000000000, 1.000000000000000000 ) ) ;
#11747=VERTEX_POINT ( 'NONE', #6377 ) ;
#11756=EDGE_CURVE ( 'NONE', #7877, #1386, #3080, .T. ) ;
#11758=CIRCLE ( 'NONE', #2255, 2.649999999999988365 ) ;
#11767=LINE ( 'NONE', #220, #1562 ) ;
#11769=CIRCLE ( 'NONE', #13524, 9.999999999999998224 ) ;
#11777=VERTEX_POINT ( 'NONE', #2069 ) ;
#11804=CIRCLE ( 'NONE', #13337, 12.49999999999999645 ) ;
#11813=CARTESIAN_POINT ( 'NONE',  ( -62.49999999999997158, 40.00000000000001421, -9.999999999999998224 ) ) ;
#11844=VERTEX_POINT ( 'NONE', #200 ) ;
#11856=LINE ( 'NONE', #7785, #1564 ) ;
#11857=CARTESIAN_POINT ( 'NONE',  ( 62.49999999999998579, 40.00000000000001421, -5.000000000000000000 ) ) ;
#11884=VECTOR ( 'NONE', #5181, 1000.000000000000000 ) ;
#11892=ORIENTED_EDGE ( 'NONE', *, *, #3183, .T. ) ;
#11894=VERTEX_POINT ( 'NONE', #11813 ) ;
#11906=CARTESIAN_POINT ( 'NONE',  ( -62.49999999999997158, 20.00000000000001421, 9.999999999999998224 ) ) ;
#11916=CARTESIAN_POINT ( 'NONE',  ( 10.00000000000000000, 25.00000000000001776, 15.00000000000000000 ) ) ;
#11921=EDGE_CURVE ( 'NONE', #345, #10123, #1159, .T. ) ;
#11941=DIRECTION ( 'NONE',  ( 0.000000000000000000, 0.000000000000000000, -1.000000000000000000 ) ) ;
#11950=CARTESIAN_POINT ( 'NONE',  ( 0.000000000000000000, 20.00000000000001421, -9.999999999999998224 ) ) ;
#11952=DIRECTION ( 'NONE',  ( 0.000000000000000000, 0.000000000000000000, -1.000000000000000000 ) ) ;
#11960=DIRECTION ( 'NONE',  ( -0.000000000000000000, 1.000000000000000000, -0.000000000000000000 ) ) ;
#11961=EDGE_CURVE ( 'NONE', #13619, #10697, #2524, .T. ) ;
#11966=AXIS2_PLACEMENT_3D ( 'NONE', #9634, #1959, #7304 ) ;
#11972=CYLINDRICAL_SURFACE ( 'NONE', #11558, 9.999999999999998224 ) ;
#12007=CARTESIAN_POINT ( 'NONE',  ( 62.49999999999998579, 45.00000000000001421, -15.00000000000000000 ) ) ;
#12013=VECTOR ( 'NONE', #3503, 1000.000000000000000 ) ;
#12015=EDGE_CURVE ( 'NONE', #9183, #2907, #10840, .T. ) ;
#12020=CIRCLE ( 'NONE', #3846, 9.999999999999998224 ) ;
#12026=AXIS2_PLACEMENT_3D ( 'NONE', #7921, #2802, #5921 ) ;
#12031=EDGE_CURVE ( 'NONE', #9042, #10299, #1561, .T. ) ;
#12036=CYLINDRICAL_SURFACE ( 'NONE', #6048, 2.649999999999988365 ) ;
#12045=DIRECTION ( 'NONE',  ( 1.000000000000000000, 0.000000000000000000, 0.000000000000000000 ) ) ;
#12046=CARTESIAN_POINT ( 'NONE',  ( 62.50000000000000000, 20.00000000000001421, 15.00000000000000000 ) ) ;
#12054=VERTEX_POINT ( 'NONE', #10975 ) ;
#12077=DIRECTION ( 'NONE',  ( 0.000000000000000000, 0.000000000000000000, -1.000000000000000000 ) ) ;
#12084=ORIENTED_EDGE ( 'NONE', *, *, #5017, .F. ) ;
#12096=ADVANCED_FACE ( 'NONE', ( #9048 ), #8919, .F. ) ;
#12106=DIRECTION ( 'NONE',  ( -0.000000000000000000, 1.000000000000000000, -0.000000000000000000 ) ) ;
#12109=EDGE_CURVE ( 'NONE', #345, #13190, #529, .T. ) ;
#12133=AXIS2_PLACEMENT_3D ( 'NONE', #6838, #463, #4910 ) ;
#12139=DIRECTION ( 'NONE',  ( 0.000000000000000000, 0.000000000000000000, -1.000000000000000000 ) ) ;
#12147=DIRECTION ( 'NONE',  ( -0.000000000000000000, 1.000000000000000000, -0.000000000000000000 ) ) ;
#12175=CARTESIAN_POINT ( 'NONE',  ( 75.00000000000000000, 32.50000000000001421, 15.00000000000000000 ) ) ;
#12189=ORIENTED_EDGE ( 'NONE', *, *, #11756, .T. ) ;
#12201=FACE_OUTER_BOUND ( 'NONE', #2678, .T. ) ;
#12202=VERTEX_POINT ( 'NONE', #12427 ) ;
#12216=CARTESIAN_POINT ( 'NONE',  ( 1.925929944387235853E-31, 15.00000000000001599, 15.00000000000000000 ) ) ;
#12221=ORIENTED_EDGE ( 'NONE', *, *, #2638, .F. ) ;
#12257=EDGE_LOOP ( 'NONE', ( #5789, #7725, #2402, #2871 ) ) ;
#12289=ORIENTED_EDGE ( 'NONE', *, *, #12015, .F. ) ;
#12290=ORIENTED_EDGE ( 'NONE', *, *, #11756, .F. ) ;
#12321=ORIENTED_EDGE ( 'NONE', *, *, #4901, .F. ) ;
#12329=LINE ( 'NONE', #8266, #3582 ) ;
#12343=DIRECTION ( 'NONE',  ( -1.000000000000000000, 0.000000000000000000, 0.000000000000000000 ) ) ;
#12346=PLANE ( 'NONE',  #5393 ) ;
#12347=EDGE_CURVE ( 'NONE', #245, #919, #3099, .T. ) ;
#12355=EDGE_CURVE ( 'NONE', #6754, #10018, #10288, .T. ) ;
#12360=LINE ( 'NONE', #8222, #3283 ) ;
#12372=EDGE_LOOP ( 'NONE', ( #2963, #13128, #8848, #9286 ) ) ;
#12375=CARTESIAN_POINT ( 'NONE',  ( -9.999999999999996447, 25.00000000000001776, -15.00000000000000000 ) ) ;
#12377=AXIS2_PLACEMENT_3D ( 'NONE', #3879, #6856, #6926 ) ;
#12378=FACE_OUTER_BOUND ( 'NONE', #13325, .T. ) ;
#12398=DIRECTION ( 'NONE',  ( -1.000000000000000000, 0.000000000000000000, 0.000000000000000000 ) ) ;
#12399=DIRECTION ( 'NONE',  ( -0.000000000000000000, -0.000000000000000000, 1.000000000000000000 ) ) ;
#12416=LINE ( 'NONE', #5246, #6208 ) ;
#12427=CARTESIAN_POINT ( 'NONE',  ( -9.999999999999998224, 15.00000000000001776, 15.00000000000000000 ) ) ;
#12439=CARTESIAN_POINT ( 'NONE',  ( -62.49999999999997158, 32.50000000000001421, 15.00000000000000000 ) ) ;
#12454=ORIENTED_EDGE ( 'NONE', *, *, #12355, .F. ) ;
#12468=CARTESIAN_POINT ( 'NONE',  ( -74.99999999999997158, 40.00000000000001421, -4.999999999999984013 ) ) ;
#12470=CARTESIAN_POINT ( 'NONE',  ( -62.49999999999997158, 45.00000000000001421, 15.00000000000000000 ) ) ;
#12476=VERTEX_POINT ( 'NONE', #12894 ) ;
#12514=FACE_OUTER_BOUND ( 'NONE', #1983, .T. ) ;
#12527=ORIENTED_EDGE ( 'NONE', *, *, #10320, .F. ) ;
#12536=CARTESIAN_POINT ( 'NONE',  ( 62.50000000000000000, 20.00000000000001421, -9.999999999999998224 ) ) ;
#12538=AXIS2_PLACEMENT_3D ( 'NONE', #10858, #13064, #4505 ) ;
#12548=CARTESIAN_POINT ( 'NONE',  ( -62.49999999999997158, 45.00000000000001421, 9.999999999999998224 ) ) ;
#12565=VECTOR ( 'NONE', #994, 1000.000000000000000 ) ;
#12589=EDGE_CURVE ( 'NONE', #9920, #2907, #1210, .T. ) ;
#12594=VERTEX_POINT ( 'NONE', #12007 ) ;
#12597=EDGE_CURVE ( 'NONE', #7922, #12594, #9861, .T. ) ;
#12600=EDGE_CURVE ( 'NONE', #10838, #7994, #7851, .T. ) ;
#12605=CARTESIAN_POINT ( 'NONE',  ( 1.925929944387235853E-31, 15.00000000000001599, 9.999999999999998224 ) ) ;
#12614=CARTESIAN_POINT ( 'NONE',  ( 2.649999999999988809, 15.00000000000001599, -15.00000000000000000 ) ) ;
#12617=CIRCLE ( 'NONE', #12822, 12.49999999999999645 ) ;
#12636=VECTOR ( 'NONE', #499, 1000.000000000000000 ) ;
#12641=CARTESIAN_POINT ( 'NONE',  ( 62.49999999999998579, 32.50000000000001421, -15.00000000000000000 ) ) ;
#12649=DIRECTION ( 'NONE',  ( 1.000000000000000000, 0.000000000000000000, 0.000000000000000000 ) ) ;
#12668=DIRECTION ( 'NONE',  ( -0.000000000000000000, -0.000000000000000000, 1.000000000000000000 ) ) ;
#12680=CARTESIAN_POINT ( 'NONE',  ( 62.49999999999998579, 40.00000000000001421, -9.999999999999998224 ) ) ;
#12682=EDGE_CURVE ( 'NONE', #12202, #5130, #7416, .T. ) ;
#12688=CARTESIAN_POINT ( 'NONE',  ( 1.925929944387235853E-31, 15.00000000000001599, -9.999999999999998224 ) ) ;
#12696=EDGE_LOOP ( 'NONE', ( #13061, #9341, #2625, #7810 ) ) ;
#12697=AXIS2_PLACEMENT_3D ( 'NONE', #2735, #1684, #5927 ) ;
#12708=ORIENTED_EDGE ( 'NONE', *, *, #9047, .F. ) ;
#12714=DIRECTION ( 'NONE',  ( 0.000000000000000000, 1.000000000000000000, 0.000000000000000000 ) ) ;
#12746=EDGE_CURVE ( 'NONE', #4573, #9060, #11383, .T. ) ;
#12753=ORIENTED_EDGE ( 'NONE', *, *, #4811, .F. ) ;
#12773=ORIENTED_EDGE ( 'NONE', *, *, #12109, .F. ) ;
#12793=LINE ( 'NONE', #10726, #9935 ) ;
#12800=CARTESIAN_POINT ( 'NONE',  ( 10.00000000000000000, 15.00000000000001776, 15.00000000000000000 ) ) ;
#12809=CARTESIAN_POINT ( 'NONE',  ( 9.999999999999994671, 20.00000000000001421, 15.00000000000000000 ) ) ;
#12821=ORIENTED_EDGE ( 'NONE', *, *, #8983, .T. ) ;
#12822=AXIS2_PLACEMENT_3D ( 'NONE', #8071, #2737, #12343 ) ;
#12851=ORIENTED_EDGE ( 'NONE', *, *, #12600, .F. ) ;
#12860=DIRECTION ( 'NONE',  ( 0.000000000000000000, 0.000000000000000000, -1.000000000000000000 ) ) ;
#12887=VERTEX_POINT ( 'NONE', #12680 ) ;
#12894=CARTESIAN_POINT ( 'NONE',  ( 10.00000000000000000, 20.00000000000001421, 15.00000000000000000 ) ) ;
#12896=DIRECTION ( 'NONE',  ( -0.000000000000000000, -0.000000000000000000, 1.000000000000000000 ) ) ;
#12899=VECTOR ( 'NONE', #8910, 1000.000000000000000 ) ;
#12908=ORIENTED_EDGE ( 'NONE', *, *, #1200, .F. ) ;
#12923=CARTESIAN_POINT ( 'NONE',  ( 1.925929944387235853E-31, 15.00000000000001599, 15.00000000000000000 ) ) ;
#12926=PLANE ( 'NONE',  #11630 ) ;
#12942=DIRECTION ( 'NONE',  ( -1.000000000000000000, 0.000000000000000000, 0.000000000000000000 ) ) ;
#12945=EDGE_CURVE ( 'NONE', #8787, #9119, #9511, .T. ) ;
#12969=VECTOR ( 'NONE', #10233, 1000.000000000000000 ) ;
#12984=LINE ( 'NONE', #7754, #11102 ) ;
#12994=DIRECTION ( 'NONE',  ( -1.000000000000000000, 0.000000000000000000, 0.000000000000000000 ) ) ;
#13016=MECHANICAL_DESIGN_GEOMETRIC_PRESENTATION_REPRESENTATION('',(#648),#8416);
#13024=VERTEX_POINT ( 'NONE', #9711 ) ;
#13038=DIRECTION ( 'NONE',  ( 0.000000000000000000, 1.000000000000000000, 0.000000000000000000 ) ) ;
#13055=CIRCLE ( 'NONE', #9107, 12.49999999999999645 ) ;
#13057=VECTOR ( 'NONE', #5990, 1000.000000000000000 ) ;
#13058=ORIENTED_EDGE ( 'NONE', *, *, #12597, .F. ) ;
#13061=ORIENTED_EDGE ( 'NONE', *, *, #7162, .T. ) ;
#13064=DIRECTION ( 'NONE',  ( -0.000000000000000000, 0.000000000000000000, -1.000000000000000000 ) ) ;
#13067=CYLINDRICAL_SURFACE ( 'NONE', #9570, 2.649999999999985700 ) ;
#13079=AXIS2_PLACEMENT_3D ( 'NONE', #7722, #244, #6687 ) ;
#13084=CLOSED_SHELL ( 'NONE', ( #2217, #1080, #4952, #2675, #7939, #10907, #266, #10244, #8409, #6569, #3801, #9657, #2052, #7667, #4148, #10832, #7647, #6855, #5663, #8509, #1195, #10970, #13469, #12096, #94, #157, #1022, #8928, #960, #97, #3567, #1618, #4469, #5528, #3488, #4498, #7478, #6716 ) ) ;
#13094=ORIENTED_EDGE ( 'NONE', *, *, #4677, .T. ) ;
#13095=FACE_OUTER_BOUND ( 'NONE', #5633, .T. ) ;
#13105=CARTESIAN_POINT ( 'NONE',  ( 62.49999999999998579, 5.000000000000018652, 5.000000000000000000 ) ) ;
#13108=CARTESIAN_POINT ( 'NONE',  ( -74.99999999999997158, 20.00000000000001421, 15.00000000000000000 ) ) ;
#13128=ORIENTED_EDGE ( 'NONE', *, *, #4202, .T. ) ;
#13132=VECTOR ( 'NONE', #5375, 1000.000000000000000 ) ;
#13135=LINE ( 'NONE', #351, #4878 ) ;
#13159=EDGE_LOOP ( 'NONE', ( #13058, #6015, #3533, #7881 ) ) ;
#13160=DIRECTION ( 'NONE',  ( 0.000000000000000000, 0.000000000000000000, -1.000000000000000000 ) ) ;
#13164=CARTESIAN_POINT ( 'NONE',  ( 62.49999999999998579, 32.50000000000001421, 15.00000000000000000 ) ) ;
#13168=LINE ( 'NONE', #7934, #5859 ) ;
#13174=ORIENTED_EDGE ( 'NONE', *, *, #3217, .F. ) ;
#13178=DIRECTION ( 'NONE',  ( -0.000000000000000000, 0.000000000000000000, -1.000000000000000000 ) ) ;
#13190=VERTEX_POINT ( 'NONE', #7911 ) ;
#13193=SHAPE_REPRESENTATION_RELATIONSHIP ( 'NONE' , 'NONE' ,  #3897, #1529 ) ;
#13194=DIRECTION ( 'NONE',  ( 0.000000000000000000, 0.000000000000000000, -1.000000000000000000 ) ) ;
#13203=ORIENTED_EDGE ( 'NONE', *, *, #1323, .F. ) ;
#13209=DIRECTION ( 'NONE',  ( 0.000000000000000000, -0.000000000000000000, 1.000000000000000000 ) ) ;
#13255=ORIENTED_EDGE ( 'NONE', *, *, #4540, .F. ) ;
#13259=VERTEX_POINT ( 'NONE', #4661 ) ;
#13264=DIRECTION ( 'NONE',  ( 0.000000000000000000, 0.000000000000000000, -1.000000000000000000 ) ) ;
#13266=CARTESIAN_POINT ( 'NONE',  ( -74.99999999999997158, 45.00000000000001421, 15.00000000000000000 ) ) ;
#13288=DIRECTION ( 'NONE',  ( -1.000000000000000000, 0.000000000000000000, 1.224646799147353207E-16 ) ) ;
#13294=EDGE_LOOP ( 'NONE', ( #12708, #10902, #6511, #6656 ) ) ;
#13295=EDGE_LOOP ( 'NONE', ( #9674, #8880 ) ) ;
#13298=CARTESIAN_POINT ( 'NONE',  ( -62.49999999999997158, 32.50000000000001421, -15.00000000000000000 ) ) ;
#13302=FACE_OUTER_BOUND ( 'NONE', #8347, .T. ) ;
#13320=LINE ( 'NONE', #8236, #490 ) ;
#13325=EDGE_LOOP ( 'NONE', ( #7390, #3497, #3518, #10474 ) ) ;
#13326=ORIENTED_EDGE ( 'NONE', *, *, #11678, .T. ) ;
#13332=CARTESIAN_POINT ( 'NONE',  ( 32.49999999999998579, 40.00000000000001421, 15.00000000000000000 ) ) ;
#13337=AXIS2_PLACEMENT_3D ( 'NONE', #516, #6971, #8970 ) ;
#13356=CARTESIAN_POINT ( 'NONE',  ( 1.925929944387235853E-31, 15.00000000000001599, -9.999999999999998224 ) ) ;
#13374=CARTESIAN_POINT ( 'NONE',  ( 0.000000000000000000, 20.00000000000001421, 9.999999999999998224 ) ) ;
#13377=ORIENTED_EDGE ( 'NONE', *, *, #4599, .T. ) ;
#13414=EDGE_CURVE ( 'NONE', #10018, #4781, #12020, .T. ) ;
#13469=ADVANCED_FACE ( 'NONE', ( #219, #4437, #4307 ), #7489, .T. ) ;
#13474=DIRECTION ( 'NONE',  ( 0.000000000000000000, 0.000000000000000000, -1.000000000000000000 ) ) ;
#13492=CARTESIAN_POINT ( 'NONE',  ( 1.925929944387235853E-31, 15.00000000000001599, 15.00000000000000000 ) ) ;
#13501=VECTOR ( 'NONE', #13288, 1000.000000000000000 ) ;
#13507=CARTESIAN_POINT ( 'NONE',  ( -2.649999999999988365, 15.00000000000001599, 15.00000000000000000 ) ) ;
#13508=CARTESIAN_POINT ( 'NONE',  ( -74.99999999999997158, 40.00000000000001421, 15.00000000000000000 ) ) ;
#13511=DIRECTION ( 'NONE',  ( 0.000000000000000000, 0.000000000000000000, -1.000000000000000000 ) ) ;
#13522=EDGE_CURVE ( 'NONE', #10854, #10505, #2218, .T. ) ;
#13524=AXIS2_PLACEMENT_3D ( 'NONE', #11477, #10438, #2832 ) ;
#13555=ORIENTED_EDGE ( 'NONE', *, *, #533, .F. ) ;
#13557=AXIS2_PLACEMENT_3D ( 'NONE', #8663, #12860, #10459 ) ;
#13561=VECTOR ( 'NONE', #4757, 1000.000000000000000 ) ;
#13619=VERTEX_POINT ( 'NONE', #10597 ) ;
#13622=CARTESIAN_POINT ( 'NONE',  ( 10.00000000000000000, 25.00000000000001776, 15.00000000000000000 ) ) ;
#13656=ORIENTED_EDGE ( 'NONE', *, *, #10484, .F. ) ;
#13660=DIRECTION ( 'NONE',  ( -1.000000000000000000, 0.000000000000000000, 1.224646799147353207E-16 ) ) ;
#13692=COLOUR_RGB('Sky Blue',0.24,0.69,0.87);
#13693=FILL_AREA_STYLE_COLOUR('',#13692);
#13694=FILL_AREA_STYLE('',(#13693));
#13695=SURFACE_STYLE_FILL_AREA(#13694);
#13696=SURFACE_SIDE_STYLE('',(#13695));
#13697=SURFACE_STYLE_USAGE(.BOTH.,#13696);
#13698=PRESENTATION_STYLE_ASSIGNMENT((#13697));
ENDSEC;
END-ISO-10303-21;
